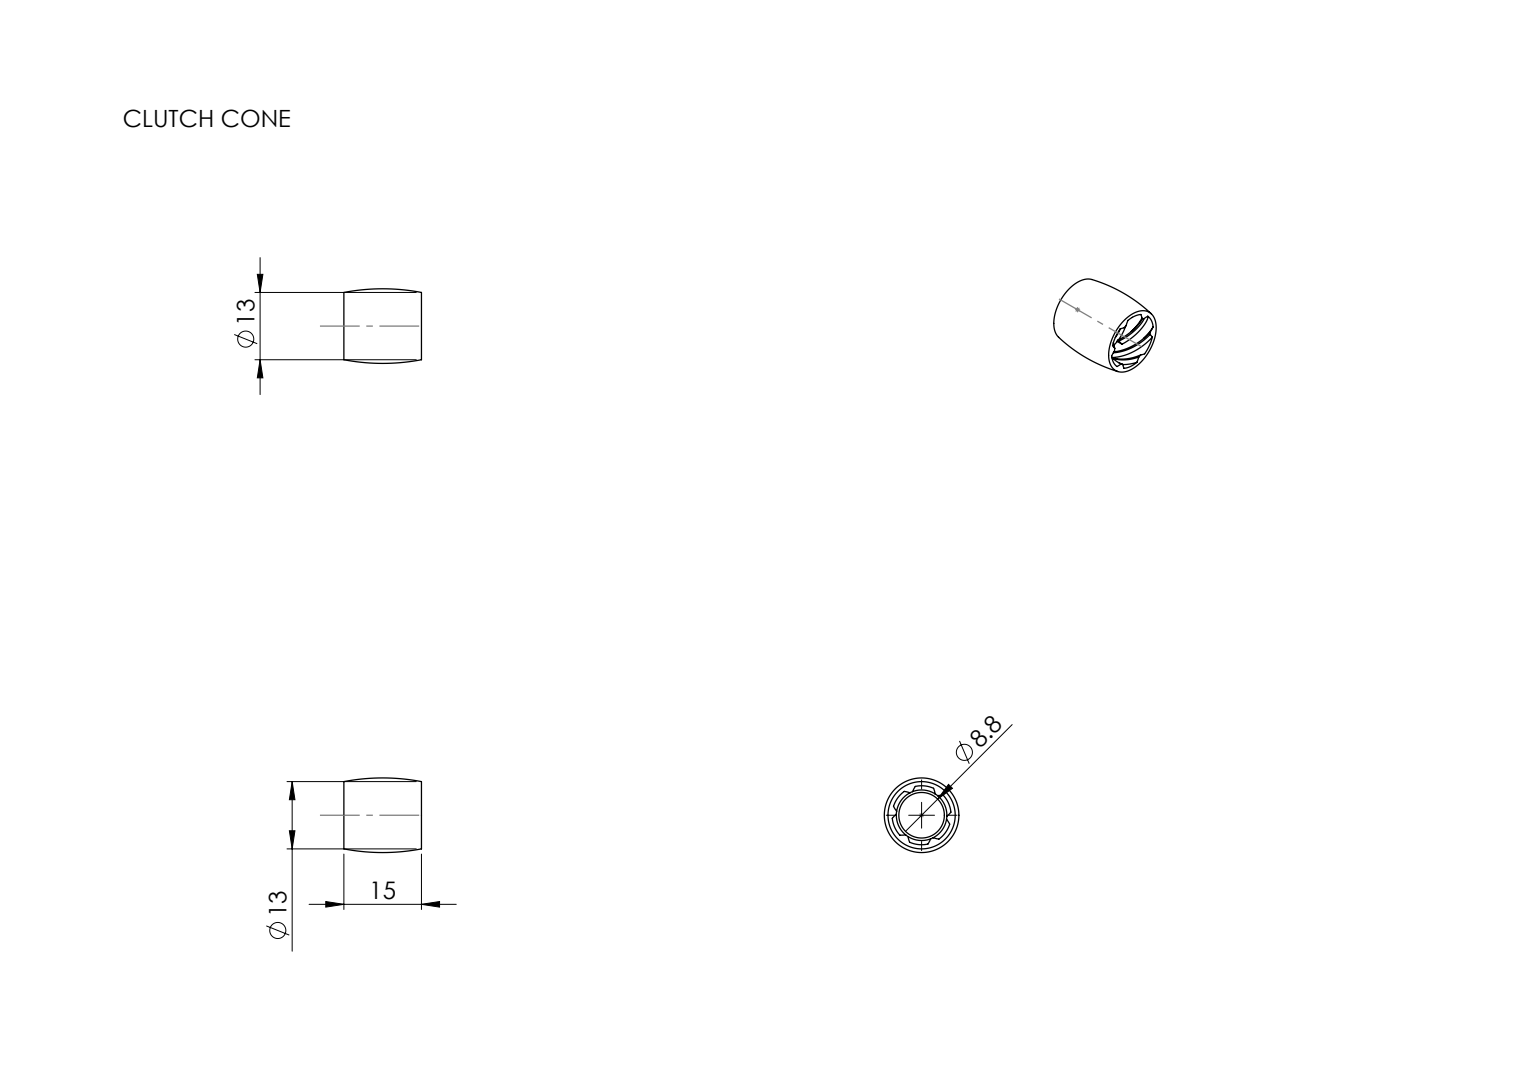
ISO-10303-21;
HEADER;
FILE_DESCRIPTION (('STEP AP214'),
    '1' );
FILE_NAME ('CLUTCH CONE.step',
    '2026-10-08T05:56:58',
    ( '' ),
    ( '' ),
    'SwSTEP 2.0',
    'SolidWorks 2026',
    '' );
FILE_SCHEMA (( 'AUTOMOTIVE_DESIGN' ));
ENDSEC;

DATA;
#4=FACE_OUTER_BOUND ( 'NONE', #5916, .T. ) ;
#7=CARTESIAN_POINT ( 'NONE',  ( 9.343749997951615427, -3.499494075959840966, 3.499494075959791672 ) ) ;
#8=EDGE_CURVE ( 'NONE', #13643, #9700, #6131, .T. ) ;
#15=VERTEX_POINT ( 'NONE', #17446 ) ;
#18=CARTESIAN_POINT ( 'NONE',  ( 12.84374999795161543, 1.016293382781411792, 4.781284448697195266 ) ) ;
#56=CARTESIAN_POINT ( 'NONE',  ( 12.34374999795161543, 4.888101187500000222, 0.7741991708318884946 ) ) ;
#57=ORIENTED_EDGE ( 'NONE', *, *, #11077, .F. ) ;
#63=CIRCLE ( 'NONE', #5149, 40.00000000000000711 ) ;
#70=ORIENTED_EDGE ( 'NONE', *, *, #8344, .T. ) ;
#73=DIRECTION ( 'NONE',  ( -1.000000000000000000, 0.000000000000000000, 0.000000000000000000 ) ) ;
#91=CARTESIAN_POINT ( 'NONE',  ( 13.34374999795161365, -0.2590123213420631454, -4.942249507334558700 ) ) ;
#94=CARTESIAN_POINT ( 'NONE',  ( 8.468749997951615427, -1.988169868018530462, -4.465502636338051445 ) ) ;
#100=AXIS2_PLACEMENT_3D ( 'NONE', #5188, #8093, #8295 ) ;
#103=CARTESIAN_POINT ( 'NONE',  ( -2.000000000000001776, 3.950217066951266176, 3.681818181818181213 ) ) ;
#104=CARTESIAN_POINT ( 'NONE',  ( 11.46874999795161543, -2.444050593750019651, 4.233219804643871598 ) ) ;
#105=CARTESIAN_POINT ( 'NONE',  ( 10.50000000000000711, 3.631840208645794821, 4.484949146646379781 ) ) ;
#106=FACE_OUTER_BOUND ( 'NONE', #19772, .T. ) ;
#139=AXIS2_PLACEMENT_3D ( 'NONE', #2060, #12472, #13976 ) ;
#145=ORIENTED_EDGE ( 'NONE', *, *, #8344, .F. ) ;
#146=CARTESIAN_POINT ( 'NONE',  ( 13.00000000000000533, 0.5958122406256767256, -5.668774803599153422 ) ) ;
#147=CARTESIAN_POINT ( 'NONE',  ( 10.34374999795161543, 0.2590123213421660631, -4.942249507334553371 ) ) ;
#148=ORIENTED_EDGE ( 'NONE', *, *, #16940, .F. ) ;
#156=( BOUNDED_SURFACE ( )  B_SPLINE_SURFACE ( 1, 2, ( 
 ( #19696, #12102, #10210, #2584, #16407, #18204, #1100, #2682, #8800, #7272, #189, #18685, #7680, #9499, #382, #3485, #10992 ),
 ( #15499, #9592, #10894, #9295, #13794, #4787, #17096, #10700, #6275, #4590, #15690, #10794, #17000, #15330, #18396, #284, #6461 ) ),
 .UNSPECIFIED., .F., .F., .F. ) 
 B_SPLINE_SURFACE_WITH_KNOTS ( ( 2, 2 ),
 ( 3, 2, 2, 2, 2, 2, 2, 2, 3 ),
 ( 0.000000000000000000, 1.000000000000000000 ),
 ( 0.000000000000000000, 0.05000000000000000278, 0.1000000000000000056, 0.1499999999999999944, 0.2000000000000000111, 0.2500000000000000000, 0.2999999999999999889, 0.3499999999999999778, 0.4000000000000000222 ),
 .UNSPECIFIED. ) 
 GEOMETRIC_REPRESENTATION_ITEM ( )  RATIONAL_B_SPLINE_SURFACE ( (
 ( 1.000000000000000000, 0.9876883405951377704, 1.000000000000000000, 0.9876883405951377704, 1.000000000000000000, 0.9876883405951377704, 1.000000000000000000, 0.9876883405951377704, 1.000000000000000000, 0.9876883405951377704, 1.000000000000000000, 0.9876883405951377704, 1.000000000000000000, 0.9876883405951377704, 1.000000000000000000, 0.9876883405951377704, 1.000000000000000000),
 ( 1.000000000000000000, 0.9876883405951377704, 1.000000000000000000, 0.9876883405951377704, 1.000000000000000000, 0.9876883405951377704, 1.000000000000000000, 0.9876883405951377704, 1.000000000000000000, 0.9876883405951377704, 1.000000000000000000, 0.9876883405951377704, 1.000000000000000000, 0.9876883405951377704, 1.000000000000000000, 0.9876883405951377704, 1.000000000000000000) ) ) 
 REPRESENTATION_ITEM ( '' )  SURFACE ( )  );
#174=EDGE_CURVE ( 'NONE', #16744, #5554, #14796, .T. ) ;
#175=CARTESIAN_POINT ( 'NONE',  ( 6.234374998975811266, 0.000000000000000000, -5.294050593750000644 ) ) ;
#186=CARTESIAN_POINT ( 'NONE',  ( 7.843749997951614539, -3.270778111535287191, -3.632567103900569361 ) ) ;
#189=CARTESIAN_POINT ( 'NONE',  ( 11.46874999795161543, 2.444050593750049405, -4.233219804643852946 ) ) ;
#193=AXIS2_PLACEMENT_3D ( 'NONE', #6002, #12326, #18419 ) ;
#203=CARTESIAN_POINT ( 'NONE',  ( 13.46874999795161543, -4.465502636338038123, 1.988169868018562880 ) ) ;
#210=CARTESIAN_POINT ( 'NONE',  ( -2.000000000000001776, 3.218695387886217674, 2.999999999999999556 ) ) ;
#211=AXIS2_PLACEMENT_3D ( 'NONE', #17804, #14615, #6883 ) ;
#213=CARTESIAN_POINT ( 'NONE',  ( 14.84374999795161543, -2.873153789725797935, -3.954556930911881096 ) ) ;
#243=CARTESIAN_POINT ( 'NONE',  ( 8.843749997951615427, -1.988169868018530462, -4.465502636338051445 ) ) ;
#252=CARTESIAN_POINT ( 'NONE',  ( 11.46874999795161543, 2.444050593749990785, 4.233219804643887585 ) ) ;
#284=CARTESIAN_POINT ( 'NONE',  ( 13.50000000000000533, 5.574407415329178939, -1.493657965219446382 ) ) ;
#289=CARTESIAN_POINT ( 'NONE',  ( 2.999999999999998224, -2.487173708821168283, 2.318181818181817455 ) ) ;
#299=CARTESIAN_POINT ( 'NONE',  ( 7.312499995903225525, 4.936344801571308061, -2.849999999999989431 ) ) ;
#308=CARTESIAN_POINT ( 'NONE',  ( 8.500000000000005329, -1.493657965219446160, -5.574407415329178939 ) ) ;
#320=ORIENTED_EDGE ( 'NONE', *, *, #14476, .T. ) ;
#343=CYLINDRICAL_SURFACE ( 'NONE', #4937, 5.400000000000000355 ) ;
#345=CARTESIAN_POINT ( 'NONE',  ( 6.843749997951615427, -3.413342815706642518E-14, 4.888101187500000222 ) ) ;
#346=CARTESIAN_POINT ( 'NONE',  ( 14.34374999795161365, -1.280903732194453859, 4.780397808154257078 ) ) ;
#379=CARTESIAN_POINT ( 'NONE',  ( 7.343749997951615427, -0.7741991708319229115, 4.888101187499994893 ) ) ;
#381=ORIENTED_EDGE ( 'NONE', *, *, #16041, .F. ) ;
#382=CARTESIAN_POINT ( 'NONE',  ( 13.46874999795161543, 4.465502636338051445, -1.988169868018530906 ) ) ;
#400=CARTESIAN_POINT ( 'NONE',  ( 6.468749997951615427, 4.233219804643887585, -2.444050593749990341 ) ) ;
#406=EDGE_LOOP ( 'NONE', ( #6297, #10419, #12416, #16842 ) ) ;
#407=CARTESIAN_POINT ( 'NONE',  ( 12.84374999795161543, -4.648860486681943627, -1.510506337161893642 ) ) ;
#416=CARTESIAN_POINT ( 'NONE',  ( 7.312499995903225525, 0.000000000000000000, -5.700000000000001066 ) ) ;
#418=PLANE ( 'NONE',  #2750 ) ;
#448=CARTESIAN_POINT ( 'NONE',  ( 10.31249999590322552, -0.5958122406255588199, -5.668774803599165857 ) ) ;
#463=CARTESIAN_POINT ( 'NONE',  ( 8.968749997951613651, 1.280903732194420996, 4.780397808154265960 ) ) ;
#485=CARTESIAN_POINT ( 'NONE',  ( 12.46874999795161543, 3.632567103900569361, -3.270778111535288080 ) ) ;
#494=DIRECTION ( 'NONE',  ( 0.000000000000000000, 0.7315216790650493905, -0.6818181818181815457 ) ) ;
#496=CARTESIAN_POINT ( 'NONE',  ( 6.843749997951615427, 4.233219804643887585, -2.444050593749990785 ) ) ;
#509=CARTESIAN_POINT ( 'NONE',  ( 14.46874999795161720, -1.988169868018592856, 4.465502636338025688 ) ) ;
#534=EDGE_LOOP ( 'NONE', ( #18812, #9374, #9796, #10381, #12618, #14253, #16988, #12583 ) ) ;
#545=VECTOR ( 'NONE', #19579, 1000.000000000000000 ) ;
#554=CARTESIAN_POINT ( 'NONE',  ( 11.84374999795161365, 2.444050593750049405, -4.233219804643852946 ) ) ;
#555=CARTESIAN_POINT ( 'NONE',  ( 9.343749997951615427, 1.280903732194420996, 4.780397808154265960 ) ) ;
#560=FACE_OUTER_BOUND ( 'NONE', #8813, .T. ) ;
#564=CARTESIAN_POINT ( 'NONE',  ( 9.165444847914525184, 0.2987243419133224775, 5.700000000000001954 ) ) ;
#566=CARTESIAN_POINT ( 'NONE',  ( 9.968749997951615427, -0.2590123213421313686, 4.942249507334556036 ) ) ;
#582=CARTESIAN_POINT ( 'NONE',  ( -2.000000000000001776, 3.950217066951266176, 3.681818181818181213 ) ) ;
#588=DIRECTION ( 'NONE',  ( -1.000000000000000000, -0.000000000000000000, -0.000000000000000000 ) ) ;
#593=CARTESIAN_POINT ( 'NONE',  ( 6.656249997951614539, 4.233219804643887585, -2.444050593749990341 ) ) ;
#603=UNCERTAINTY_MEASURE_WITH_UNIT (LENGTH_MEASURE( 1.000000000000000082E-05 ), #7664, 'distance_accuracy_value', 'NONE');
#606=CARTESIAN_POINT ( 'NONE',  ( 11.46874999795161543, -2.444050593749961031, -4.233219804643904460 ) ) ;
#611=CARTESIAN_POINT ( 'NONE',  ( 11.50000000000000355, 3.631840208645857437, -4.484949146646330931 ) ) ;
#618=CARTESIAN_POINT ( 'NONE',  ( 11.31249999590322375, 5.421022142882375938, -1.761396867937200739 ) ) ;
#624=CARTESIAN_POINT ( 'NONE',  ( 6.968749997951614539, -0.7741991708319229115, 4.888101187499994893 ) ) ;
#629=FACE_BOUND ( 'NONE', #5913, .T. ) ;
#653=CARTESIAN_POINT ( 'NONE',  ( 8.843749997951615427, 1.988169868018562436, 4.465502636338039011 ) ) ;
#654=CARTESIAN_POINT ( 'NONE',  ( 14.46874999795161720, -1.988169868018592856, 4.465502636338025688 ) ) ;
#659=CARTESIAN_POINT ( 'NONE',  ( 13.00000000000000000, -4.125339889944092953, 2.622041954598548941 ) ) ;
#660=EDGE_CURVE ( 'NONE', #13507, #7007, #3581, .T. ) ;
#664=CIRCLE ( 'NONE', #18238, 5.700000000000001954 ) ;
#668=CARTESIAN_POINT ( 'NONE',  ( 13.46874999795161543, 0.5109457054262118714, -4.861323657744403448 ) ) ;
#675=( LENGTH_UNIT ( ) NAMED_UNIT ( * ) SI_UNIT ( .MILLI., .METRE. ) );
#682=EDGE_LOOP ( 'NONE', ( #3661, #6850, #15777, #2392 ) ) ;
#685=CARTESIAN_POINT ( 'NONE',  ( 13.00000000000000178, -4.444590484536226960, -2.035510078342938733 ) ) ;
#703=EDGE_CURVE ( 'NONE', #2779, #5327, #19540, .T. ) ;
#704=FACE_OUTER_BOUND ( 'NONE', #6201, .T. ) ;
#710=PLANE ( 'NONE',  #13946 ) ;
#713=EDGE_CURVE ( 'NONE', #18575, #7007, #1785, .T. ) ;
#720=VERTEX_POINT ( 'NONE', #3211 ) ;
#752=ORIENTED_EDGE ( 'NONE', *, *, #660, .F. ) ;
#754=CARTESIAN_POINT ( 'NONE',  ( 13.00000000000000178, -4.920309236097862637, -1.604440756441545268 ) ) ;
#762=CARTESIAN_POINT ( 'NONE',  ( 12.65441706489329299, -5.699999999999998401, -0.6173595171471657483 ) ) ;
#781=CARTESIAN_POINT ( 'NONE',  ( 12.66727757604273386, -4.360680574150373717E-16, 5.700000000000001066 ) ) ;
#794=CARTESIAN_POINT ( 'NONE',  ( 10.34374999795161543, -4.150607464521772094, -2.695436003842760719 ) ) ;
#795=CARTESIAN_POINT ( 'NONE',  ( 9.312499995903225525, 2.318398865532038666, 5.207209108562838473 ) ) ;
#800=CIRCLE ( 'NONE', #3027, 6.500000000000002665 ) ;
#802=UNCERTAINTY_MEASURE_WITH_UNIT (LENGTH_MEASURE( 1.000000000000000082E-05 ), #13780, 'distance_accuracy_value', 'NONE');
#804=CARTESIAN_POINT ( 'NONE',  ( 13.84374999795161543, 0.5109457054262118714, -4.861323657744403448 ) ) ;
#808=LINE ( 'NONE', #16007, #5368 ) ;
#863=CARTESIAN_POINT ( 'NONE',  ( 7.000000000000005329, -1.761396867937238486, 5.421022142882364392 ) ) ;
#871=VERTEX_POINT ( 'NONE', #14621 ) ;
#878=CARTESIAN_POINT ( 'NONE',  ( 13.00000000000000178, -3.869963285057273605, 2.986818217332043446 ) ) ;
#887=CARTESIAN_POINT ( 'NONE',  ( 11.34374999795161543, 3.114526743279256049, 3.846120219227944670 ) ) ;
#897=AXIS2_PLACEMENT_3D ( 'NONE', #9316, #9724, #10914 ) ;
#902=CARTESIAN_POINT ( 'NONE',  ( 9.343749997951615427, -3.499494075959840966, 3.499494075959791672 ) ) ;
#914=EDGE_CURVE ( 'NONE', #11016, #5140, #8465, .T. ) ;
#917=( BOUNDED_CURVE ( )  B_SPLINE_CURVE ( 2, ( #9368, #13668, #1364, #16672, #9267, #19759, #1464, #6048, #12170, #18270, #4558, #56, #6149, #16875, #15372 ),
 .UNSPECIFIED., .F., .F. ) 
 B_SPLINE_CURVE_WITH_KNOTS ( ( 3, 2, 2, 2, 2, 2, 2, 3 ),
 ( 0.000000000000000000, 0.05000000000000000278, 0.1000000000000000056, 0.1499999999999999944, 0.2000000000000000111, 0.2500000000000000000, 0.2999999999999999889, 0.3078686208676164604 ),
 .UNSPECIFIED. ) 
 CURVE ( )  GEOMETRIC_REPRESENTATION_ITEM ( )  RATIONAL_B_SPLINE_CURVE ( ( 1.000000000000000000, 0.9876883405951377704, 1.000000000000000000, 0.9876883405951377704, 1.000000000000000000, 0.9876883405951377704, 1.000000000000000000, 0.9876883405951377704, 1.000000000000000000, 0.9876883405951377704, 1.000000000000000000, 0.9876883405951377704, 1.000000000000000000, 0.9980624843978382899, 0.9967347918236166837 ) ) 
 REPRESENTATION_ITEM ( '' )  );
#918=CARTESIAN_POINT ( 'NONE',  ( 9.312499995903225525, -5.668774803599153422, -0.5958122406256771697 ) ) ;
#939=ORIENTED_EDGE ( 'NONE', *, *, #8365, .F. ) ;
#964=CARTESIAN_POINT ( 'NONE',  ( 12.50000000000000533, -4.840010801796506890, 3.143139765844590983 ) ) ;
#976=CARTESIAN_POINT ( 'NONE',  ( 13.00000000000000178, 0.000000000000000000, 0.000000000000000000 ) ) ;
#979=EDGE_CURVE ( 'NONE', #11644, #4794, #11939, .T. ) ;
#1002=DIRECTION ( 'NONE',  ( 0.000000000000000000, 0.4999999999999920619, 0.8660254037844432595 ) ) ;
#1011=DIRECTION ( 'NONE',  ( -1.000000000000000000, 0.000000000000000000, 0.000000000000000000 ) ) ;
#1037=CARTESIAN_POINT ( 'NONE',  ( 11.96874999795161365, -3.114526743279282250, 3.846120219227923798 ) ) ;
#1067=CARTESIAN_POINT ( 'NONE',  ( 11.00000000000000711, -2.850000000000023626, 4.936344801571289409 ) ) ;
#1080=CARTESIAN_POINT ( 'NONE',  ( 12.84374999795161543, 4.648860486681953397, 1.510506337161861223 ) ) ;
#1081=CARTESIAN_POINT ( 'NONE',  ( 9.343749997951615427, 4.780397808154257078, 1.280903732194454081 ) ) ;
#1100=CARTESIAN_POINT ( 'NONE',  ( 9.468749997951615427, -0.5109457054261099529, -4.861323657744413218 ) ) ;
#1110=CARTESIAN_POINT ( 'NONE',  ( 10.00000000000000533, -5.421022142882388373, 1.761396867937162769 ) ) ;
#1114=CARTESIAN_POINT ( 'NONE',  ( 9.468749997951615427, -3.954556930911881985, 2.873153789725797491 ) ) ;
#1136=CARTESIAN_POINT ( 'NONE',  ( 13.00000000000000000, 1.727010089215937905, 5.432074755721460591 ) ) ;
#1139=CARTESIAN_POINT ( 'NONE',  ( 7.968749997951616315, 2.695436003842704764, 4.150607464521812062 ) ) ;
#1145=CARTESIAN_POINT ( 'NONE',  ( 8.500000000000007105, -5.574407415329147852, -1.493657965219562511 ) ) ;
#1148=EDGE_CURVE ( 'NONE', #5529, #11664, #6279, .T. ) ;
#1150=ADVANCED_FACE ( 'NONE', ( #6371 ), #5472, .F. ) ;
#1165=CARTESIAN_POINT ( 'NONE',  ( 11.50000000000000355, -3.631840208645826351, 4.484949146646356688 ) ) ;
#1166=CIRCLE ( 'NONE', #11076, 6.500000000000000000 ) ;
#1177=CARTESIAN_POINT ( 'NONE',  ( 11.31249999590322375, 5.421022142882375938, -1.761396867937200739 ) ) ;
#1184=DIRECTION ( 'NONE',  ( -1.000000000000000000, -0.000000000000000000, -0.000000000000000000 ) ) ;
#1190=CARTESIAN_POINT ( 'NONE',  ( 12.99999999999999467, 4.496324317583058949, 1.917446440021246756 ) ) ;
#1198=LINE ( 'NONE', #9203, #10258 ) ;
#1211=CARTESIAN_POINT ( 'NONE',  ( 12.84374999795161543, 4.648860486681953397, 1.510506337161861223 ) ) ;
#1217=CARTESIAN_POINT ( 'NONE',  ( 11.31249999590322375, -1.185096637661254171, 5.575441324182689229 ) ) ;
#1236=CARTESIAN_POINT ( 'NONE',  ( 11.46874999795161543, -2.444050593749961031, -4.233219804643904460 ) ) ;
#1247=EDGE_CURVE ( 'NONE', #19695, #4381, #18662, .T. ) ;
#1253=CARTESIAN_POINT ( 'NONE',  ( 12.73273607671833929, -0.6164700669140440459, -4.866269517993464078 ) ) ;
#1263=CARTESIAN_POINT ( 'NONE',  ( 9.000000000000005329, 0.5958122406255991210, 5.668774803599163192 ) ) ;
#1270=EDGE_LOOP ( 'NONE', ( #9959, #8302, #10280, #10813 ) ) ;
#1275=CARTESIAN_POINT ( 'NONE',  ( -2.000000000000001776, -3.950217066951263956, -3.681818181818183877 ) ) ;
#1293=CARTESIAN_POINT ( 'NONE',  ( 7.343749997951615427, 3.846120219227923798, 3.114526743279282694 ) ) ;
#1297=CARTESIAN_POINT ( 'NONE',  ( 13.00000000000000178, 0.000000000000000000, 0.000000000000000000 ) ) ;
#1298=CARTESIAN_POINT ( 'NONE',  ( 12.00000000000000533, 1.185096637661215757, 5.575441324182695446 ) ) ;
#1300=CARTESIAN_POINT ( 'NONE',  ( 11.46874999795161543, 4.888101187500000222, -2.993098736590125853E-16 ) ) ;
#1305=CARTESIAN_POINT ( 'NONE',  ( 13.00000000000000000, -1.727010089215899713, -5.432074755721473025 ) ) ;
#1306=EDGE_LOOP ( 'NONE', ( #18307, #12651, #14806, #1467 ) ) ;
#1309=CARTESIAN_POINT ( 'NONE',  ( 9.343749997951615427, 3.499494075959816541, -3.499494075959816541 ) ) ;
#1312=CARTESIAN_POINT ( 'NONE',  ( 6.234374998975811266, -3.696815770993907903E-14, 5.294050593750000644 ) ) ;
#1319=CARTESIAN_POINT ( 'NONE',  ( -2.000000000000001776, 0.000000000000000000, 0.000000000000000000 ) ) ;
#1323=DIRECTION ( 'NONE',  ( 0.000000000000000000, 0.000000000000000000, 1.000000000000000000 ) ) ;
#1324=CARTESIAN_POINT ( 'NONE',  ( 11.96874999795161365, 4.888101187500000222, 0.7741991708318884946 ) ) ;
#1333=CARTESIAN_POINT ( 'NONE',  ( 14.46874999795161720, 1.988169868018623720, -4.465502636338010589 ) ) ;
#1334=VECTOR ( 'NONE', #5423, 1000.000000000000000 ) ;
#1347=CIRCLE ( 'NONE', #4219, 5.400000000000000355 ) ;
#1351=ADVANCED_FACE ( 'NONE', ( #10582 ), #7915, .F. ) ;
#1359=DIRECTION ( 'NONE',  ( -1.000000000000000000, 0.000000000000000000, 0.000000000000000000 ) ) ;
#1364=CARTESIAN_POINT ( 'NONE',  ( 7.843749997951614539, 1.510506337161861445, -4.648860486681953397 ) ) ;
#1370=AXIS2_PLACEMENT_3D ( 'NONE', #6319, #18637, #4934 ) ;
#1375=COLOUR_RGB ( '', 0.31764706, 0.68627451, 0.89019608) ;
#1388=PRODUCT_DEFINITION_CONTEXT ( 'detailed design', #10473, 'design' ) ;
#1398=ORIENTED_EDGE ( 'NONE', *, *, #1665, .T. ) ;
#1399=CARTESIAN_POINT ( 'NONE',  ( 11.34374999795161543, -1.773574444220757274, 4.620319390059819398 ) ) ;
#1402=AXIS2_PLACEMENT_3D ( 'NONE', #15006, #10704, #16607 ) ;
#1404=CARTESIAN_POINT ( 'NONE',  ( 10.50000000000000533, 3.631840208645794821, 4.484949146646379781 ) ) ;
#1408=DIRECTION ( 'NONE',  ( 0.000000000000000000, 0.000000000000000000, 1.000000000000000000 ) ) ;
#1427=CARTESIAN_POINT ( 'NONE',  ( 8.812499995903225525, 5.763142191869157216, -0.3020334839682480288 ) ) ;
#1438=CARTESIAN_POINT ( 'NONE',  ( 8.000000000000005329, -5.668774803599153422, -0.5958122406256771697 ) ) ;
#1442=( BOUNDED_CURVE ( )  B_SPLINE_CURVE ( 2, ( #19181, #2085, #15798, #15900, #795, #5474, #11300, #3588, #8495 ),
 .UNSPECIFIED., .F., .F. ) 
 B_SPLINE_CURVE_WITH_KNOTS ( ( 3, 2, 2, 2, 3 ),
 ( 0.000000000000000000, 0.04999999999999999584, 0.09999999999999999167, 0.1499999999999999944, 0.1666819079834116757 ),
 .UNSPECIFIED. ) 
 CURVE ( )  GEOMETRIC_REPRESENTATION_ITEM ( )  RATIONAL_B_SPLINE_CURVE ( ( 1.000000000000000000, 0.9876883405951377704, 1.000000000000000000, 0.9876883405951377704, 1.000000000000000000, 0.9876883405951377704, 1.000000000000000000, 0.9958923606136996787, 0.9945256517182512468 ) ) 
 REPRESENTATION_ITEM ( '' )  );
#1443=EDGE_CURVE ( 'NONE', #3546, #9343, #18377, .T. ) ;
#1446=CARTESIAN_POINT ( 'NONE',  ( 13.00000000000000178, 3.849641071994447383, -3.458892414715164065 ) ) ;
#1464=CARTESIAN_POINT ( 'NONE',  ( 9.843749997951615427, 3.954556930911862000, -2.873153789725825469 ) ) ;
#1467=ORIENTED_EDGE ( 'NONE', *, *, #6341, .F. ) ;
#1468=EDGE_CURVE ( 'NONE', #11673, #18486, #18038, .T. ) ;
#1473=CARTESIAN_POINT ( 'NONE',  ( 9.812499995903223748, 4.080749450109650844, -4.080749450109650844 ) ) ;
#1494=CARTESIAN_POINT ( 'NONE',  ( 12.34374999795161543, -3.114526743279282250, 3.846120219227923798 ) ) ;
#1497=CARTESIAN_POINT ( 'NONE',  ( -2.000000000000001776, 0.000000000000000000, 0.000000000000000000 ) ) ;
#1498=CARTESIAN_POINT ( 'NONE',  ( 12.33180101230371584, 0.5990941410143489909, 5.700000000000001066 ) ) ;
#1499=EDGE_CURVE ( 'NONE', #871, #3717, #6504, .T. ) ;
#1501=ORIENTED_EDGE ( 'NONE', *, *, #11729, .T. ) ;
#1507=CARTESIAN_POINT ( 'NONE',  ( 12.65441706489329299, -2.315350974882445456, -5.245024560144885939 ) ) ;
#1513=CARTESIAN_POINT ( 'NONE',  ( 12.46874999795161543, 4.648860486681953397, 1.510506337161861223 ) ) ;
#1517=ORIENTED_EDGE ( 'NONE', *, *, #3744, .F. ) ;
#1527=CARTESIAN_POINT ( 'NONE',  ( 9.312499995903225525, 5.668774803599156975, 0.5958122406256377568 ) ) ;
#1528=CARTESIAN_POINT ( 'NONE',  ( 13.00000000000000000, 4.333424887443004359, 2.261628166637590365 ) ) ;
#1538=CARTESIAN_POINT ( 'NONE',  ( 9.968749997951615427, 4.150607464521791634, 2.695436003842732298 ) ) ;
#1549=DIRECTION ( 'NONE',  ( -1.000000000000000000, -0.000000000000000000, -0.000000000000000000 ) ) ;
#1555=EDGE_CURVE ( 'NONE', #5021, #2350, #12018, .T. ) ;
#1569=CARTESIAN_POINT ( 'NONE',  ( 7.843749997951614539, 3.270778111535313837, 3.632567103900546712 ) ) ;
#1593=CARTESIAN_POINT ( 'NONE',  ( 6.500000000000005329, 5.387740456496234565, -2.068159791354182708 ) ) ;
#1595=EDGE_LOOP ( 'NONE', ( #18905, #4122 ) ) ;
#1596=CARTESIAN_POINT ( 'NONE',  ( 8.500000000000007105, 4.080749450109650844, -4.080749450109650844 ) ) ;
#1611=CARTESIAN_POINT ( 'NONE',  ( 9.968749997951617203, -4.409619785863921670, 2.246813503491803310 ) ) ;
#1620=CARTESIAN_POINT ( 'NONE',  ( 10.96874999795161720, 4.888101187500000222, -0.7741991708318890497 ) ) ;
#1630=DIRECTION ( 'NONE',  ( -1.000000000000000000, 0.000000000000000000, 0.000000000000000000 ) ) ;
#1631=CARTESIAN_POINT ( 'NONE',  ( 11.96874999795161365, 1.773574444220725299, 4.620319390059829168 ) ) ;
#1638=APPLICATION_CONTEXT ( 'automotive_design' ) ;
#1645=CARTESIAN_POINT ( 'NONE',  ( 9.343749997951615427, -1.280903732194386579, -4.780397808154273953 ) ) ;
#1647=ORIENTED_EDGE ( 'NONE', *, *, #11077, .T. ) ;
#1665=EDGE_CURVE ( 'NONE', #18575, #9272, #2209, .T. ) ;
#1669=CARTESIAN_POINT ( 'NONE',  ( 13.00000000000000178, -0.7793280607714923036, -4.825575716215948496 ) ) ;
#1718=ORIENTED_EDGE ( 'NONE', *, *, #4065, .T. ) ;
#1722=CARTESIAN_POINT ( 'NONE',  ( 13.00000000000000000, 5.567819778318904511, 1.220402768007685657 ) ) ;
#1736=CARTESIAN_POINT ( 'NONE',  ( 13.00000000000000000, 0.2080849974989116558, 4.883670121236158401 ) ) ;
#1747=CARTESIAN_POINT ( 'NONE',  ( 11.81249999590322552, 2.068159791354259092, -5.387740456496206143 ) ) ;
#1755=CARTESIAN_POINT ( 'NONE',  ( 12.84374999795161543, 1.016293382781411792, 4.781284448697194378 ) ) ;
#1785=( BOUNDED_CURVE ( )  B_SPLINE_CURVE ( 2, ( #416, #3613, #6496, #12425, #15721, #12625, #17320, #14321, #618, #6694, #3511, #17222, #11325 ),
 .UNSPECIFIED., .F., .F. ) 
 B_SPLINE_CURVE_WITH_KNOTS ( ( 3, 2, 2, 2, 2, 2, 3 ),
 ( 0.000000000000000000, 0.05000000000000000278, 0.1000000000000000056, 0.1499999999999999944, 0.2000000000000000111, 0.2500000000000000000, 0.2843253191101273170 ),
 .UNSPECIFIED. ) 
 CURVE ( )  GEOMETRIC_REPRESENTATION_ITEM ( )  RATIONAL_B_SPLINE_CURVE ( ( 1.000000000000000000, 0.9876883405951377704, 1.000000000000000000, 0.9876883405951377704, 1.000000000000000000, 0.9876883405951377704, 1.000000000000000000, 0.9876883405951377704, 1.000000000000000000, 0.9876883405951377704, 1.000000000000000000, 0.9915479672430580482, 0.9947006833465674713 ) ) 
 REPRESENTATION_ITEM ( '' )  );
#1786=CARTESIAN_POINT ( 'NONE',  ( 9.843749997951615427, -4.465502636338009701, -1.988169868018624609 ) ) ;
#1800=CARTESIAN_POINT ( 'NONE',  ( 9.000000000000005329, 5.207209108562820710, 2.318398865532074193 ) ) ;
#1809=CARTESIAN_POINT ( 'NONE',  ( 11.46874999795161543, -4.888101187500000222, -3.383411828340740850E-14 ) ) ;
#1815=EDGE_LOOP ( 'NONE', ( #19167, #8420, #70, #12884 ) ) ;
#1852=CARTESIAN_POINT ( 'NONE',  ( 8.843749997951615427, 4.861323657744407001, 0.5109457054261784537 ) ) ;
#1853=VERTEX_POINT ( 'NONE', #14815 ) ;
#1876=CARTESIAN_POINT ( 'NONE',  ( 12.99999999999999467, 4.057257337410506537, -2.726922038711639740 ) ) ;
#1878=EDGE_LOOP ( 'NONE', ( #6627, #4972, #13147, #5239, #9251 ) ) ;
#1884=CARTESIAN_POINT ( 'NONE',  ( 11.34374999795161543, -3.114526743279228072, -3.846120219227966430 ) ) ;
#1903=DIRECTION ( 'NONE',  ( 0.000000000000000000, 0.000000000000000000, -1.000000000000000000 ) ) ;
#1937=CARTESIAN_POINT ( 'NONE',  ( 14.31249999590322552, 5.207209108562852684, -2.318398865532001363 ) ) ;
#1943=CARTESIAN_POINT ( 'NONE',  ( 12.96874999795161543, 0.2590123213420971182, 4.942249507334556924 ) ) ;
#1973=ORIENTED_EDGE ( 'NONE', *, *, #10065, .T. ) ;
#1974=CARTESIAN_POINT ( 'NONE',  ( 13.34374999795161365, 4.150607464521828938, -2.695436003842674566 ) ) ;
#2000=ORIENTED_EDGE ( 'NONE', *, *, #14470, .F. ) ;
#2006=CARTESIAN_POINT ( 'NONE',  ( 11.00000000000000711, 2.850000000000057820, -4.936344801571268093 ) ) ;
#2028=VERTEX_POINT ( 'NONE', #13504 ) ;
#2038=CARTESIAN_POINT ( 'NONE',  ( 10.81249999590322375, 0.3020334839683282979, -5.763142191869152775 ) ) ;
#2039=CARTESIAN_POINT ( 'NONE',  ( 13.00000000000000178, -0.7156116249825553721, -4.835865888676779356 ) ) ;
#2046=CARTESIAN_POINT ( 'NONE',  ( 6.000000000000005329, 0.000000000000000000, 0.000000000000000000 ) ) ;
#2060=CARTESIAN_POINT ( 'NONE',  ( 13.00000000000000178, 4.400000000000000355, 0.000000000000000000 ) ) ;
#2075=( BOUNDED_CURVE ( )  B_SPLINE_CURVE ( 2, ( #3081, #19596, #10698 ),
 .UNSPECIFIED., .F., .F. ) 
 B_SPLINE_CURVE_WITH_KNOTS ( ( 3, 3 ),
 ( 0.3333180920165871863, 0.3500000000000000333 ),
 .UNSPECIFIED. ) 
 CURVE ( )  GEOMETRIC_REPRESENTATION_ITEM ( )  RATIONAL_B_SPLINE_CURVE ( ( 0.9945256517182510247, 0.9958923606136993456, 1.000000000000000000 ) ) 
 REPRESENTATION_ITEM ( '' )  );
#2079=CARTESIAN_POINT ( 'NONE',  ( 9.000000000000005329, 4.611396867937201272, -3.350375938067097437 ) ) ;
#2085=CARTESIAN_POINT ( 'NONE',  ( 7.812499995903224637, 4.484949146646356688, 3.631840208645826795 ) ) ;
#2094=CARTESIAN_POINT ( 'NONE',  ( 10.96874999795161720, -1.773574444220757274, 4.620319390059819398 ) ) ;
#2101=CARTESIAN_POINT ( 'NONE',  ( 9.843749997951615427, -3.954556930911881985, 2.873153789725797491 ) ) ;
#2143=ORIENTED_EDGE ( 'NONE', *, *, #2952, .T. ) ;
#2144=CARTESIAN_POINT ( 'NONE',  ( 6.468749997951615427, 4.233219804643887585, -2.444050593749990341 ) ) ;
#2159=VECTOR ( 'NONE', #8743, 1000.000000000000000 ) ;
#2164=DIRECTION ( 'NONE',  ( -1.000000000000000000, -0.000000000000000000, -0.000000000000000000 ) ) ;
#2169=CARTESIAN_POINT ( 'NONE',  ( 12.99999999999999467, 3.985098679772364427, -2.831373229855470797 ) ) ;
#2174=CARTESIAN_POINT ( 'NONE',  ( 8.468749997951615427, -1.988169868018530462, -4.465502636338051445 ) ) ;
#2175=CARTESIAN_POINT ( 'NONE',  ( 12.31249999590322552, 2.850000000000057820, -4.936344801571268093 ) ) ;
#2184=CARTESIAN_POINT ( 'NONE',  ( -2.000000000000001776, 0.000000000000000000, 0.000000000000000000 ) ) ;
#2195=CARTESIAN_POINT ( 'NONE',  ( 13.84374999795161543, -3.954556930911842016, -2.873153789725852558 ) ) ;
#2209=LINE ( 'NONE', #18820, #15168 ) ;
#2211=CARTESIAN_POINT ( 'NONE',  ( 6.468749997951615427, -3.413342815706642518E-14, 4.888101187500000222 ) ) ;
#2243=CARTESIAN_POINT ( 'NONE',  ( 13.34374999795161365, -4.150607464521812062, 2.695436003842704764 ) ) ;
#2264=VECTOR ( 'NONE', #14846, 1000.000000000000114 ) ;
#2265=FILL_AREA_STYLE_COLOUR ( '', #1375 ) ;
#2274=CARTESIAN_POINT ( 'NONE',  ( 7.968749997951616315, -2.695436003842674566, -4.150607464521828938 ) ) ;
#2275=CARTESIAN_POINT ( 'NONE',  ( 9.843749997951615427, -0.5109457054261099529, -4.861323657744413218 ) ) ;
#2279=CARTESIAN_POINT ( 'NONE',  ( 10.50000000000000533, 5.700000000000000178, -0.9027913098498572264 ) ) ;
#2292=CARTESIAN_POINT ( 'NONE',  ( 8.843749997951615427, -4.861323657744403448, -0.5109457054262123155 ) ) ;
#2297=CARTESIAN_POINT ( 'NONE',  ( 12.00000000000000533, 4.235925505221192822, -3.814044456245444081 ) ) ;
#2306=ORIENTED_EDGE ( 'NONE', *, *, #1555, .T. ) ;
#2314=DIRECTION ( 'NONE',  ( 1.000000000000000000, 0.000000000000000000, 0.000000000000000000 ) ) ;
#2350=VERTEX_POINT ( 'NONE', #19088 ) ;
#2357=PLANE ( 'NONE',  #12766 ) ;
#2363=SURFACE_STYLE_USAGE ( .BOTH. , #12875 ) ;
#2371=CARTESIAN_POINT ( 'NONE',  ( 12.34374999795161543, 3.114526743279308896, -3.846120219227901593 ) ) ;
#2372=CARTESIAN_POINT ( 'NONE',  ( 11.31249999590322375, 1.185096637661293251, -5.575441324182679459 ) ) ;
#2384=CARTESIAN_POINT ( 'NONE',  ( 10.81249999590322375, 4.840010801796482909, 3.143139765844622957 ) ) ;
#2385=CIRCLE ( 'NONE', #18054, 5.400000000000000355 ) ;
#2389=CARTESIAN_POINT ( 'NONE',  ( 10.34374999795161543, -4.150607464521772094, -2.695436003842760275 ) ) ;
#2392=ORIENTED_EDGE ( 'NONE', *, *, #6340, .F. ) ;
#2393=CARTESIAN_POINT ( 'NONE',  ( 15.31249999590322552, -3.350375938067065906, -4.611396867937224364 ) ) ;
#2417=DIRECTION ( 'NONE',  ( 0.000000000000000000, 0.000000000000000000, 1.000000000000000000 ) ) ;
#2422=AXIS2_PLACEMENT_3D ( 'NONE', #19522, #10438, #1323 ) ;
#2442=ORIENTED_EDGE ( 'NONE', *, *, #14853, .T. ) ;
#2445=CARTESIAN_POINT ( 'NONE',  ( 13.00000000000000533, -4.611396867937178179, -3.350375938067128967 ) ) ;
#2451=FILL_AREA_STYLE ('',( #2265 ) ) ;
#2456=CARTESIAN_POINT ( 'NONE',  ( 9.968749997951617203, -0.2590123213421313686, 4.942249507334556036 ) ) ;
#2461=CARTESIAN_POINT ( 'NONE',  ( 6.843749997951615427, -4.233219804643852946, -2.444050593750049849 ) ) ;
#2476=CARTESIAN_POINT ( 'NONE',  ( 11.31249999590322375, 4.235925505221138643, 3.814044456245502701 ) ) ;
#2480=EDGE_CURVE ( 'NONE', #18417, #2569, #18920, .T. ) ;
#2485=DIRECTION ( 'NONE',  ( 1.000000000000000000, 0.000000000000000000, 0.000000000000000000 ) ) ;
#2490=CARTESIAN_POINT ( 'NONE',  ( -2.000000000000001776, 5.388445916248354013E-16, -4.400000000000000355 ) ) ;
#2530=CARTESIAN_POINT ( 'NONE',  ( -2.000000000000001776, 0.000000000000000000, 0.000000000000000000 ) ) ;
#2533=CARTESIAN_POINT ( 'NONE',  ( 9.000000000000005329, 0.5958122406255991210, 5.668774803599163192 ) ) ;
#2536=EDGE_CURVE ( 'NONE', #5021, #18417, #18673, .T. ) ;
#2541=DIRECTION ( 'NONE',  ( -1.000000000000000000, -0.000000000000000000, -0.000000000000000000 ) ) ;
#2554=FACE_OUTER_BOUND ( 'NONE', #14176, .T. ) ;
#2555=ORIENTED_EDGE ( 'NONE', *, *, #18715, .T. ) ;
#2559=CARTESIAN_POINT ( 'NONE',  ( 7.312499995903225525, -4.936344801571268093, -2.850000000000058265 ) ) ;
#2569=VERTEX_POINT ( 'NONE', #11075 ) ;
#2584=CARTESIAN_POINT ( 'NONE',  ( 7.968749997951616315, -2.695436003842674566, -4.150607464521828938 ) ) ;
#2607=CARTESIAN_POINT ( 'NONE',  ( 2.999999999999998224, 0.000000000000000000, 0.000000000000000000 ) ) ;
#2627=CARTESIAN_POINT ( 'NONE',  ( 2.999999999999998224, 3.950217066951266176, 3.681818181818181213 ) ) ;
#2631=CARTESIAN_POINT ( 'NONE',  ( 2.999999999999998224, -3.950217066951263956, -3.681818181818183877 ) ) ;
#2632=ORIENTED_EDGE ( 'NONE', *, *, #10042, .T. ) ;
#2634=MANIFOLD_SOLID_BREP ( 'Cut-Extrude-Thin1', #18032 ) ;
#2650=ORIENTED_EDGE ( 'NONE', *, *, #14058, .F. ) ;
#2660=VERTEX_POINT ( 'NONE', #18973 ) ;
#2681=EDGE_LOOP ( 'NONE', ( #14546, #4895, #5342, #15515 ) ) ;
#2682=CARTESIAN_POINT ( 'NONE',  ( 9.968749997951617203, 0.2590123213421660631, -4.942249507334553371 ) ) ;
#2685=CARTESIAN_POINT ( 'NONE',  ( 8.312499995903225525, -5.575441324182703440, 1.185096637661176677 ) ) ;
#2686=CARTESIAN_POINT ( 'NONE',  ( 13.00000000000000178, 0.000000000000000000, 6.500000000000002665 ) ) ;
#2688=EDGE_CURVE ( 'NONE', #16413, #17466, #13505, .T. ) ;
#2700=CARTESIAN_POINT ( 'NONE',  ( 9.968749997951617203, 4.409619785863906571, -2.246813503491833508 ) ) ;
#2703=ORIENTED_EDGE ( 'NONE', *, *, #713, .T. ) ;
#2706=DIRECTION ( 'NONE',  ( -1.000000000000000000, 0.000000000000000000, 0.000000000000000000 ) ) ;
#2709=( BOUNDED_CURVE ( )  B_SPLINE_CURVE ( 2, ( #9967, #15865, #18957, #11646, #16253, #19245, #8551, #6837, #14465, #17561, #11365, #762, #14660 ),
 .UNSPECIFIED., .F., .F. ) 
 B_SPLINE_CURVE_WITH_KNOTS ( ( 3, 2, 2, 2, 2, 2, 3 ),
 ( 0.000000000000000000, 0.05000000000000000278, 0.1000000000000000056, 0.1499999999999999944, 0.2000000000000000111, 0.2500000000000000000, 0.2843253191101272614 ),
 .UNSPECIFIED. ) 
 CURVE ( )  GEOMETRIC_REPRESENTATION_ITEM ( )  RATIONAL_B_SPLINE_CURVE ( ( 1.000000000000000000, 0.9876883405951377704, 1.000000000000000000, 0.9876883405951377704, 1.000000000000000000, 0.9876883405951377704, 1.000000000000000000, 0.9876883405951377704, 1.000000000000000000, 0.9876883405951377704, 1.000000000000000000, 0.9915479672430580482, 0.9947006833465674713 ) ) 
 REPRESENTATION_ITEM ( '' )  );
#2716=FACE_OUTER_BOUND ( 'NONE', #11184, .T. ) ;
#2717=CARTESIAN_POINT ( 'NONE',  ( 11.84374999795161365, -2.444050593750019651, 4.233219804643871598 ) ) ;
#2728=CARTESIAN_POINT ( 'NONE',  ( 7.500000000000005329, -5.763142191869158992, 0.3020334839682081163 ) ) ;
#2729=DIRECTION ( 'NONE',  ( 0.000000000000000000, 0.7315216790650492795, 0.6818181818181815457 ) ) ;
#2730=VERTEX_POINT ( 'NONE', #8864 ) ;
#2750=AXIS2_PLACEMENT_3D ( 'NONE', #17427, #1002, #14528 ) ;
#2751=CARTESIAN_POINT ( 'NONE',  ( 7.968749997951616315, 2.695436003842704764, 4.150607464521812062 ) ) ;
#2756=ORIENTED_EDGE ( 'NONE', *, *, #12082, .T. ) ;
#2759=EDGE_LOOP ( 'NONE', ( #5210, #19294, #7443, #4978 ) ) ;
#2764=CARTESIAN_POINT ( 'NONE',  ( 13.84374999795161543, 3.954556930911862000, 2.873153789725825025 ) ) ;
#2778=AXIS2_PLACEMENT_3D ( 'NONE', #14754, #13058, #2729 ) ;
#2779=VERTEX_POINT ( 'NONE', #4953 ) ;
#2784=CARTESIAN_POINT ( 'NONE',  ( 8.843749997951615427, 1.988169868018562436, 4.465502636338039011 ) ) ;
#2786=CARTESIAN_POINT ( 'NONE',  ( 6.656249997951614539, 4.936344801571289409, 2.850000000000024070 ) ) ;
#2787=CARTESIAN_POINT ( 'NONE',  ( 13.00000000000000000, 4.125339889944109828, -2.622041954598519187 ) ) ;
#2794=CARTESIAN_POINT ( 'NONE',  ( 14.46874999795161720, -2.873153789725797935, -3.954556930911881096 ) ) ;
#2797=ORIENTED_EDGE ( 'NONE', *, *, #12498, .T. ) ;
#2799=DIRECTION ( 'NONE',  ( 0.000000000000000000, 5.329070518200751394E-15, 1.000000000000000000 ) ) ;
#2801=ADVANCED_FACE ( 'NONE', ( #18363 ), #16964, .F. ) ;
#2803=CARTESIAN_POINT ( 'NONE',  ( 12.99999999999998046, -4.467995623377355230, -2.612285395956023493 ) ) ;
#2817=EDGE_LOOP ( 'NONE', ( #12909, #6116, #11935, #9643 ) ) ;
#2820=AXIS2_PLACEMENT_3D ( 'NONE', #5950, #18174, #8662 ) ;
#2821=CARTESIAN_POINT ( 'NONE',  ( 6.468749997951615427, 4.233219804643871598, 2.444050593750020095 ) ) ;
#2823=CARTESIAN_POINT ( 'NONE',  ( 6.656249997951614539, -3.980288726281172656E-14, 5.700000000000001066 ) ) ;
#2827=CARTESIAN_POINT ( 'NONE',  ( 12.99999999999999112, 4.467995623377368553, 2.612285395955995515 ) ) ;
#2857=CARTESIAN_POINT ( 'NONE',  ( 13.00000000000000533, -5.207209108562836697, 2.318398865532038666 ) ) ;
#2859=VERTEX_POINT ( 'NONE', #345 ) ;
#2863=DIRECTION ( 'NONE',  ( -0.000000000000000000, 0.8660254037844329345, 0.5000000000000097700 ) ) ;
#2865=CARTESIAN_POINT ( 'NONE',  ( 9.343749997951615427, 3.499494075959816541, -3.499494075959816541 ) ) ;
#2884=CARTESIAN_POINT ( 'NONE',  ( 12.84374999795161543, -3.632567103900546712, 3.270778111535314281 ) ) ;
#2887=CARTESIAN_POINT ( 'NONE',  ( 11.46874999795161543, 2.444050593750049405, -4.233219804643852946 ) ) ;
#2896=DIRECTION ( 'NONE',  ( 0.000000000000000000, 0.000000000000000000, 1.000000000000000000 ) ) ;
#2911=CARTESIAN_POINT ( 'NONE',  ( 15.31249999590322552, -2.318398865532073305, 5.207209108562820710 ) ) ;
#2923=CARTESIAN_POINT ( 'NONE',  ( 10.96874999795161720, -3.114526743279228072, -3.846120219227966430 ) ) ;
#2924=VECTOR ( 'NONE', #15921, 1000.000000000000227 ) ;
#2926=CARTESIAN_POINT ( 'NONE',  ( 12.73273607671833929, 0.6164700669140775746, 4.866269517993460525 ) ) ;
#2929=FACE_OUTER_BOUND ( 'NONE', #10183, .T. ) ;
#2952=EDGE_CURVE ( 'NONE', #5462, #12828, #11482, .T. ) ;
#2971=ORIENTED_EDGE ( 'NONE', *, *, #9449, .T. ) ;
#2974=ORIENTED_EDGE ( 'NONE', *, *, #12220, .F. ) ;
#2984=ADVANCED_FACE ( 'NONE', ( #4041 ), #18155, .F. ) ;
#2988=CARTESIAN_POINT ( 'NONE',  ( 8.343749997951611874, 2.695436003842704764, 4.150607464521812062 ) ) ;
#2991=DIRECTION ( 'NONE',  ( 0.000000000000000000, 0.000000000000000000, 1.000000000000000000 ) ) ;
#3001=CARTESIAN_POINT ( 'NONE',  ( 11.96874999795161365, -4.888101187499994893, -0.7741991708319226895 ) ) ;
#3002=CARTESIAN_POINT ( 'NONE',  ( 14.34374999795161365, 3.499494075959816541, 3.499494075959815653 ) ) ;
#3016=CARTESIAN_POINT ( 'NONE',  ( 9.343749997951615427, 4.780397808154257078, 1.280903732194454081 ) ) ;
#3026=CARTESIAN_POINT ( 'NONE',  ( 9.968749997951617203, -4.150607464521772094, -2.695436003842760275 ) ) ;
#3027=AXIS2_PLACEMENT_3D ( 'NONE', #12052, #18154, #6128 ) ;
#3028=CARTESIAN_POINT ( 'NONE',  ( 12.46874999795161543, 1.016293382781411792, 4.781284448697194378 ) ) ;
#3031=CARTESIAN_POINT ( 'NONE',  ( 2.999999999999998224, 0.000000000000000000, 0.000000000000000000 ) ) ;
#3045=CARTESIAN_POINT ( 'NONE',  ( 9.968749997951615427, -4.150607464521772094, -2.695436003842760719 ) ) ;
#3054=ORIENTED_EDGE ( 'NONE', *, *, #14618, .T. ) ;
#3060=ADVANCED_FACE ( 'NONE', ( #6286 ), #12413, .T. ) ;
#3065=( BOUNDED_CURVE ( )  B_SPLINE_CURVE ( 2, ( #7755, #14363, #12763, #6838, #8155, #463, #14056, #566, #14262, #12861, #6536, #11366, #6635, #14466, #659 ),
 .UNSPECIFIED., .F., .F. ) 
 B_SPLINE_CURVE_WITH_KNOTS ( ( 3, 2, 2, 2, 2, 2, 2, 3 ),
 ( 0.000000000000000000, 0.05000000000000000278, 0.1000000000000000056, 0.1499999999999999944, 0.2000000000000000111, 0.2500000000000000000, 0.2999999999999999889, 0.3265529187307101844 ),
 .UNSPECIFIED. ) 
 CURVE ( )  GEOMETRIC_REPRESENTATION_ITEM ( )  RATIONAL_B_SPLINE_CURVE ( ( 1.000000000000000000, 0.9876883405951377704, 1.000000000000000000, 0.9876883405951377704, 1.000000000000000000, 0.9876883405951377704, 1.000000000000000000, 0.9876883405951377704, 1.000000000000000000, 0.9876883405951377704, 1.000000000000000000, 0.9876883405951377704, 1.000000000000000000, 0.9934617901676502383, 0.9938679225082089896 ) ) 
 REPRESENTATION_ITEM ( '' )  );
#3069=VERTEX_POINT ( 'NONE', #8739 ) ;
#3081=CARTESIAN_POINT ( 'NONE',  ( 12.66727757604273386, -4.360680574150373717E-16, 5.700000000000001066 ) ) ;
#3089=CARTESIAN_POINT ( 'NONE',  ( 7.968749997951616315, -2.695436003842674122, -4.150607464521828938 ) ) ;
#3092=CARTESIAN_POINT ( 'NONE',  ( 12.00000000000000533, 5.421022142882376826, 1.761396867937200073 ) ) ;
#3101=CARTESIAN_POINT ( 'NONE',  ( 9.500000000000003553, 4.840010801796480244, 3.143139765844623401 ) ) ;
#3103=CARTESIAN_POINT ( 'NONE',  ( 12.34374999795161543, 4.888101187500000222, 0.7741991708318884946 ) ) ;
#3110=CARTESIAN_POINT ( 'NONE',  ( 7.468749997951615427, -1.510506337161893864, 4.648860486681943627 ) ) ;
#3113=VECTOR ( 'NONE', #17109, 1000.000000000000114 ) ;
#3130=ADVANCED_FACE ( 'NONE', ( #7892 ), #14100, .F. ) ;
#3133=VECTOR ( 'NONE', #19416, 1000.000000000000000 ) ;
#3188=FACE_OUTER_BOUND ( 'NONE', #2681, .T. ) ;
#3191=CARTESIAN_POINT ( 'NONE',  ( 10.50000000000000711, 5.699999999999999289, -0.9027913098498572264 ) ) ;
#3206=CARTESIAN_POINT ( 'NONE',  ( 13.96874999795161365, -3.499494075959791672, -3.499494075959840078 ) ) ;
#3211=CARTESIAN_POINT ( 'NONE',  ( 2.999999999999998224, 3.950217066951266176, -3.681818181818181213 ) ) ;
#3213=ORIENTED_EDGE ( 'NONE', *, *, #9370, .T. ) ;
#3228=CARTESIAN_POINT ( 'NONE',  ( 12.99999999999999467, 0.3952618871915727916, 4.872094134945738730 ) ) ;
#3247=CARTESIAN_POINT ( 'NONE',  ( 6.843749997951615427, 4.233219804643887585, -2.444050593749990341 ) ) ;
#3256=VECTOR ( 'NONE', #6278, 1000.000000000000000 ) ;
#3265=ORIENTED_EDGE ( 'NONE', *, *, #4373, .F. ) ;
#3283=CARTESIAN_POINT ( 'NONE',  ( 8.343749997951613651, -2.246813503491864150, 4.409619785863891472 ) ) ;
#3284=ORIENTED_EDGE ( 'NONE', *, *, #9449, .F. ) ;
#3302=CARTESIAN_POINT ( 'NONE',  ( 8.968749997951611874, 4.780397808154257078, 1.280903732194454303 ) ) ;
#3309=CARTESIAN_POINT ( 'NONE',  ( 7.000000000000005329, -3.814044456245443193, -4.235925505221191933 ) ) ;
#3318=ADVANCED_FACE ( 'NONE', ( #17696 ), #3991, .F. ) ;
#3345=CARTESIAN_POINT ( 'NONE',  ( 7.500000000000005329, -5.763142191869158992, 0.3020334839682081163 ) ) ;
#3385=CARTESIAN_POINT ( 'NONE',  ( 11.34374999795161543, -4.888101187500005551, 0.7741991708318548548 ) ) ;
#3386=EDGE_LOOP ( 'NONE', ( #12658, #18758, #13143, #5921, #14658 ) ) ;
#3414=ORIENTED_EDGE ( 'NONE', *, *, #19473, .F. ) ;
#3415=LINE ( 'NONE', #8210, #2924 ) ;
#3444=CARTESIAN_POINT ( 'NONE',  ( 8.343749997951611874, -2.695436003842674566, -4.150607464521828938 ) ) ;
#3449=SHAPE_DEFINITION_REPRESENTATION ( #13226, #14878 ) ;
#3452=CARTESIAN_POINT ( 'NONE',  ( 10.96874999795161720, 3.114526743279255161, 3.846120219227944670 ) ) ;
#3481=( BOUNDED_CURVE ( )  B_SPLINE_CURVE ( 2, ( #10155, #8255, #18857, #16062, #5442, #4048, #2533, #564, #5248 ),
 .UNSPECIFIED., .F., .F. ) 
 B_SPLINE_CURVE_WITH_KNOTS ( ( 3, 2, 2, 2, 3 ),
 ( 0.000000000000000000, 0.04999999999999999584, 0.09999999999999999167, 0.1499999999999999944, 0.1666819079834116757 ),
 .UNSPECIFIED. ) 
 CURVE ( )  GEOMETRIC_REPRESENTATION_ITEM ( )  RATIONAL_B_SPLINE_CURVE ( ( 1.000000000000000000, 0.9876883405951377704, 1.000000000000000000, 0.9876883405951377704, 1.000000000000000000, 0.9876883405951377704, 1.000000000000000000, 0.9958923606136996787, 0.9945256517182512468 ) ) 
 REPRESENTATION_ITEM ( '' )  );
#3485=CARTESIAN_POINT ( 'NONE',  ( 13.96874999795161365, 4.780397808154273065, -1.280903732194386802 ) ) ;
#3499=CARTESIAN_POINT ( 'NONE',  ( 10.96874999795161720, 3.114526743279255161, 3.846120219227944670 ) ) ;
#3506=CARTESIAN_POINT ( 'NONE',  ( 12.96874999795161543, -4.409619785863891472, -2.246813503491864150 ) ) ;
#3511=CARTESIAN_POINT ( 'NONE',  ( 12.31249999590322552, 5.700000000000001066, -3.490243377569957047E-16 ) ) ;
#3525=DIRECTION ( 'NONE',  ( -0.000000000000000000, 0.6818181818181816567, 0.7315216790650493905 ) ) ;
#3537=DIRECTION ( 'NONE',  ( -1.000000000000000000, -0.000000000000000000, -0.000000000000000000 ) ) ;
#3538=CARTESIAN_POINT ( 'NONE',  ( 7.843749997951614539, -3.270778111535287191, -3.632567103900569361 ) ) ;
#3546=VERTEX_POINT ( 'NONE', #17235 ) ;
#3573=CARTESIAN_POINT ( 'NONE',  ( 12.96874999795161543, 4.150607464521828938, -2.695436003842674566 ) ) ;
#3575=CARTESIAN_POINT ( 'NONE',  ( -2.000000000000001776, 5.388445916248354013E-16, -4.400000000000000355 ) ) ;
#3581=B_SPLINE_CURVE_WITH_KNOTS ( 'NONE', 3,
 ( #9732, #12526, #6592, #1722 ),
 .UNSPECIFIED., .F., .F.,
 ( 4, 4 ),
 ( 0.000000000000000000, 0.001126652051248517921 ),
 .UNSPECIFIED. ) ;
#3587=VECTOR ( 'NONE', #17285, 1000.000000000000114 ) ;
#3588=CARTESIAN_POINT ( 'NONE',  ( 10.47794484381774538, 0.2987243419133224775, 5.700000000000001954 ) ) ;
#3598=( GEOMETRIC_REPRESENTATION_CONTEXT ( 3 ) GLOBAL_UNCERTAINTY_ASSIGNED_CONTEXT ( ( #5770 ) ) GLOBAL_UNIT_ASSIGNED_CONTEXT ( ( #675, #19164, #18876 ) ) REPRESENTATION_CONTEXT ( 'NONE', 'WORKASPACE' ) );
#3606=CARTESIAN_POINT ( 'NONE',  ( 11.81249999590322552, -5.700000000000005507, 0.9027913098498173694 ) ) ;
#3608=AXIS2_PLACEMENT_3D ( 'NONE', #5667, #7656, #2863 ) ;
#3613=CARTESIAN_POINT ( 'NONE',  ( 7.812499995903224637, 0.9027913098498568933, -5.700000000000000178 ) ) ;
#3617=CARTESIAN_POINT ( 'NONE',  ( 9.468749997951615427, -3.954556930911881985, 2.873153789725797491 ) ) ;
#3639=CARTESIAN_POINT ( 'NONE',  ( 8.312499995903225525, -3.814044456245443193, -4.235925505221191933 ) ) ;
#3644=ORIENTED_EDGE ( 'NONE', *, *, #5582, .F. ) ;
#3645=CARTESIAN_POINT ( 'NONE',  ( 6.843749997951615427, 4.233219804643871598, 2.444050593750020095 ) ) ;
#3646=CARTESIAN_POINT ( 'NONE',  ( 10.84374999795161543, 3.632567103900523620, 3.270778111535338262 ) ) ;
#3654=ORIENTED_EDGE ( 'NONE', *, *, #16122, .T. ) ;
#3661=ORIENTED_EDGE ( 'NONE', *, *, #16689, .F. ) ;
#3676=CARTESIAN_POINT ( 'NONE',  ( 8.812499995903225525, -3.143139765844555900, -4.840010801796527318 ) ) ;
#3685=DIRECTION ( 'NONE',  ( 0.000000000000000000, 0.000000000000000000, 1.000000000000000000 ) ) ;
#3694=CARTESIAN_POINT ( 'NONE',  ( 13.00000000000000533, -5.207209108562836697, 2.318398865532038666 ) ) ;
#3695=CARTESIAN_POINT ( 'NONE',  ( 8.343749997951611874, -4.942249507334558700, 0.2590123213420631454 ) ) ;
#3717=VERTEX_POINT ( 'NONE', #10038 ) ;
#3723=DIRECTION ( 'NONE',  ( 0.000000000000000000, 0.000000000000000000, -1.000000000000000000 ) ) ;
#3729=CARTESIAN_POINT ( 'NONE',  ( 6.843749997951615427, 4.233219804643887585, -2.444050593749990785 ) ) ;
#3735=ADVANCED_FACE ( 'NONE', ( #9013 ), #16627, .F. ) ;
#3744=EDGE_CURVE ( 'NONE', #16939, #7007, #4705, .T. ) ;
#3752=CARTESIAN_POINT ( 'NONE',  ( 6.000000000000005329, 0.000000000000000000, 0.000000000000000000 ) ) ;
#3756=EDGE_LOOP ( 'NONE', ( #13695, #6353, #8426, #17868, #16338, #14629 ) ) ;
#3768=EDGE_LOOP ( 'NONE', ( #11132, #10471, #6114, #17257 ) ) ;
#3776=CARTESIAN_POINT ( 'NONE',  ( 8.343749997951613651, -2.695436003842674122, -4.150607464521828938 ) ) ;
#3778=DIRECTION ( 'NONE',  ( -1.000000000000000000, 0.000000000000000000, 0.000000000000000000 ) ) ;
#3794=B_SPLINE_CURVE_WITH_KNOTS ( 'NONE', 3,
 ( #7782, #13894, #7149, #8383, #685, #11775, #6859, #8669, #17584, #17780 ),
 .UNSPECIFIED., .F., .F.,
 ( 4, 3, 3, 4 ),
 ( 0.000000000000000000, 0.0001875345074742634278, 0.0003808595644229697272, 0.0005744879655065562602 ),
 .UNSPECIFIED. ) ;
#3795=CARTESIAN_POINT ( 'NONE',  ( 9.343749997951615427, -4.780397808154247308, -1.280903732194487166 ) ) ;
#3812=EDGE_CURVE ( 'NONE', #3717, #10033, #8362, .T. ) ;
#3814=CARTESIAN_POINT ( 'NONE',  ( 13.96874999795161365, -3.499494075959791672, -3.499494075959840078 ) ) ;
#3822=CARTESIAN_POINT ( 'NONE',  ( 7.312499995903225525, 4.936344801571289409, 2.850000000000024070 ) ) ;
#3843=CARTESIAN_POINT ( 'NONE',  ( 9.343749997951615427, 1.280903732194421218, 4.780397808154266848 ) ) ;
#3854=ORIENTED_EDGE ( 'NONE', *, *, #11239, .T. ) ;
#3863=ORIENTED_EDGE ( 'NONE', *, *, #9847, .F. ) ;
#3869=CARTESIAN_POINT ( 'NONE',  ( 14.84374999795161543, 4.861323657744413218, -0.5109457054261112852 ) ) ;
#3870=CARTESIAN_POINT ( 'NONE',  ( 7.812499995903224637, -4.484949146646330931, -3.631840208645857437 ) ) ;
#3896=CARTESIAN_POINT ( 'NONE',  ( 8.843749997951615427, -2.873153789725853002, 3.954556930911842016 ) ) ;
#3902=AXIS2_PLACEMENT_3D ( 'NONE', #16015, #8418, #11512 ) ;
#3905=LINE ( 'NONE', #19016, #7737 ) ;
#3932=ORIENTED_EDGE ( 'NONE', *, *, #17857, .F. ) ;
#3946=ORIENTED_EDGE ( 'NONE', *, *, #4395, .F. ) ;
#3950=ADVANCED_FACE ( 'NONE', ( #106 ), #18668, .F. ) ;
#3958=CARTESIAN_POINT ( 'NONE',  ( 6.656249997951614539, 4.936344801571308061, -2.849999999999989431 ) ) ;
#3960=CARTESIAN_POINT ( 'NONE',  ( 0.000000000000000000, 0.000000000000000000, 5.700000000000001954 ) ) ;
#3966=PRESENTATION_STYLE_ASSIGNMENT (( #2363 ) ) ;
#3991=CYLINDRICAL_SURFACE ( 'NONE', #5207, 5.400000000000000355 ) ;
#4013=CARTESIAN_POINT ( 'NONE',  ( 11.31249999590322375, -4.235925505221111997, -3.814044456245531567 ) ) ;
#4041=FACE_OUTER_BOUND ( 'NONE', #1306, .T. ) ;
#4043=EDGE_CURVE ( 'NONE', #9272, #13507, #917, .T. ) ;
#4044=EDGE_CURVE ( 'NONE', #11866, #18865, #3065, .T. ) ;
#4048=CARTESIAN_POINT ( 'NONE',  ( 8.500000000000005329, 1.493657965219485018, 5.574407415329170057 ) ) ;
#4055=ORIENTED_EDGE ( 'NONE', *, *, #2952, .F. ) ;
#4056=CARTESIAN_POINT ( 'NONE',  ( 7.078124996927420476, -4.584782303107560963, -2.647025296875054057 ) ) ;
#4057=CARTESIAN_POINT ( 'NONE',  ( 7.312499995903225525, -4.936344801571327601, 2.849999999999954348 ) ) ;
#4065=EDGE_CURVE ( 'NONE', #18486, #4381, #15735, .T. ) ;
#4074=CARTESIAN_POINT ( 'NONE',  ( 7.343749997951615427, -3.846120219227900705, -3.114526743279308896 ) ) ;
#4083=CARTESIAN_POINT ( 'NONE',  ( 8.343749997951613651, -4.942249507334558700, 0.2590123213420630899 ) ) ;
#4089=LINE ( 'NONE', #13480, #12079 ) ;
#4118=EDGE_LOOP ( 'NONE', ( #6163, #19732, #11072, #4810, #13734 ) ) ;
#4122=ORIENTED_EDGE ( 'NONE', *, *, #8103, .T. ) ;
#4131=CARTESIAN_POINT ( 'NONE',  ( 12.92161831991541554, -3.713244971082748425, 3.181176262573032432 ) ) ;
#4138=CARTESIAN_POINT ( 'NONE',  ( 6.968749997951614539, 3.846120219227923798, 3.114526743279282694 ) ) ;
#4149=VERTEX_POINT ( 'NONE', #9775 ) ;
#4179=CARTESIAN_POINT ( 'NONE',  ( 12.34374999795161543, 1.773574444220725743, 4.620319390059829168 ) ) ;
#4190=CARTESIAN_POINT ( 'NONE',  ( 12.99999999999999467, 4.416988234087969367, 2.093740232017179181 ) ) ;
#4191=EDGE_CURVE ( 'NONE', #18200, #5529, #14946, .T. ) ;
#4193=ADVANCED_FACE ( 'NONE', ( #13256 ), #19342, .T. ) ;
#4197=CARTESIAN_POINT ( 'NONE',  ( 9.312499995903225525, 2.318398865532038666, 5.207209108562838473 ) ) ;
#4198=CARTESIAN_POINT ( 'NONE',  ( 10.81249999590322375, -4.840010801796461593, -3.143139765844656708 ) ) ;
#4207=CARTESIAN_POINT ( 'NONE',  ( 13.00000000000000533, -4.611396867937178179, -3.350375938067128967 ) ) ;
#4208=ORIENTED_EDGE ( 'NONE', *, *, #660, .T. ) ;
#4211=CARTESIAN_POINT ( 'NONE',  ( 9.968749997951615427, -4.409619785863921670, 2.246813503491803310 ) ) ;
#4219=AXIS2_PLACEMENT_3D ( 'NONE', #1497, #13397, #10703 ) ;
#4227=CARTESIAN_POINT ( 'NONE',  ( 13.00000000000000000, 4.125339889944109828, -2.622041954598519187 ) ) ;
#4258=CARTESIAN_POINT ( 'NONE',  ( 8.468749997951615427, -4.861323657744403448, -0.5109457054262123155 ) ) ;
#4265=CARTESIAN_POINT ( 'NONE',  ( 6.968749997951614539, 3.846120219227923798, 3.114526743279282694 ) ) ;
#4267=ORIENTED_EDGE ( 'NONE', *, *, #18874, .F. ) ;
#4290=CARTESIAN_POINT ( 'NONE',  ( 13.00000000000000178, 4.545788521379996006, 1.798195097859992098 ) ) ;
#4295=CARTESIAN_POINT ( 'NONE',  ( 10.31249999590322552, 0.5958122406255991210, 5.668774803599163192 ) ) ;
#4298=CARTESIAN_POINT ( 'NONE',  ( 12.73273607671833929, 3.906077990787180099, -2.967013497616978412 ) ) ;
#4299=CARTESIAN_POINT ( 'NONE',  ( 9.000000000000005329, 5.207209108562820710, 2.318398865532074193 ) ) ;
#4302=FACE_OUTER_BOUND ( 'NONE', #6234, .T. ) ;
#4311=CARTESIAN_POINT ( 'NONE',  ( 9.468749997951615427, 3.954556930911862000, -2.873153789725825469 ) ) ;
#4327=CARTESIAN_POINT ( 'NONE',  ( 12.34374999795161543, 1.773574444220725743, 4.620319390059829168 ) ) ;
#4340=CARTESIAN_POINT ( 'NONE',  ( 7.968749997951616315, -4.942249507334558700, 0.2590123213420631454 ) ) ;
#4341=CARTESIAN_POINT ( 'NONE',  ( 9.468749997951615427, 4.465502636338023912, 1.988169868018593300 ) ) ;
#4365=CARTESIAN_POINT ( 'NONE',  ( 13.50000000000000533, -5.574407415329169169, 1.493657965219485462 ) ) ;
#4372=ORIENTED_EDGE ( 'NONE', *, *, #14387, .T. ) ;
#4373=EDGE_CURVE ( 'NONE', #2730, #2350, #5794, .T. ) ;
#4376=CARTESIAN_POINT ( 'NONE',  ( 8.812499995903225525, 2.620002426024544029, -5.142044285764750811 ) ) ;
#4381=VERTEX_POINT ( 'NONE', #13842 ) ;
#4386=CARTESIAN_POINT ( 'NONE',  ( -2.000000000000001776, 3.218695387886217230, -3.000000000000000000 ) ) ;
#4395=EDGE_CURVE ( 'NONE', #4149, #6896, #5109, .T. ) ;
#4396=CARTESIAN_POINT ( 'NONE',  ( 6.968749997951614539, -3.846120219227900705, -3.114526743279308896 ) ) ;
#4397=CARTESIAN_POINT ( 'NONE',  ( 8.500000000000005329, 5.574407415329157622, 1.493657965219523875 ) ) ;
#4403=CARTESIAN_POINT ( 'NONE',  ( 14.00000000000000533, -3.350375938067065906, -4.611396867937224364 ) ) ;
#4404=EDGE_LOOP ( 'NONE', ( #8244, #6068, #17246, #145 ) ) ;
#4410=DIRECTION ( 'NONE',  ( 0.000000000000000000, 6.982962677686267499E-15, -1.000000000000000000 ) ) ;
#4418=EDGE_CURVE ( 'NONE', #6896, #10630, #19163, .T. ) ;
#4419=DIRECTION ( 'NONE',  ( 0.000000000000000000, 0.000000000000000000, 1.000000000000000000 ) ) ;
#4437=CARTESIAN_POINT ( 'NONE',  ( 13.00000000000000533, 4.560365019702147471, 2.978280878416429633 ) ) ;
#4442=DIRECTION ( 'NONE',  ( 0.000000000000000000, 0.000000000000000000, 1.000000000000000000 ) ) ;
#4453=CARTESIAN_POINT ( 'NONE',  ( 9.468749997951615427, -4.465502636338009701, -1.988169868018624609 ) ) ;
#4467=CARTESIAN_POINT ( 'NONE',  ( 6.000593838912648081, -0.002144393866035136480, 5.699999596629369059 ) ) ;
#4473=CARTESIAN_POINT ( 'NONE',  ( 6.234374998975811266, -3.696815770993907903E-14, 5.294050593750000644 ) ) ;
#4479=DIRECTION ( 'NONE',  ( 1.000000000000000000, 0.000000000000000000, 0.000000000000000000 ) ) ;
#4486=VECTOR ( 'NONE', #4479, 1000.000000000000000 ) ;
#4487=EDGE_LOOP ( 'NONE', ( #16822, #9810, #13995, #9536 ) ) ;
#4488=CARTESIAN_POINT ( 'NONE',  ( 12.31249999590322552, -2.850000000000023626, 4.936344801571289409 ) ) ;
#4491=CARTESIAN_POINT ( 'NONE',  ( 10.46874999795161720, 1.016293382781477961, -4.781284448697179279 ) ) ;
#4500=CARTESIAN_POINT ( 'NONE',  ( 7.843749997951614539, 1.510506337161861445, -4.648860486681953397 ) ) ;
#4515=CARTESIAN_POINT ( 'NONE',  ( 13.81249999590322552, 0.3020334839682480288, 5.763142191869157216 ) ) ;
#4517=EDGE_LOOP ( 'NONE', ( #13105, #6804 ) ) ;
#4538=VERTEX_POINT ( 'NONE', #3822 ) ;
#4558=CARTESIAN_POINT ( 'NONE',  ( 11.84374999795161365, 4.888101187500000222, -2.993098736590125853E-16 ) ) ;
#4568=EDGE_CURVE ( 'NONE', #720, #18915, #16032, .T. ) ;
#4571=CARTESIAN_POINT ( 'NONE',  ( 10.31249999590322552, 4.611396867937201272, -3.350375938067097437 ) ) ;
#4590=CARTESIAN_POINT ( 'NONE',  ( 10.50000000000000711, 2.068159791354259092, -5.387740456496206143 ) ) ;
#4595=AXIS2_PLACEMENT_3D ( 'NONE', #18890, #6865, #8390 ) ;
#4600=CARTESIAN_POINT ( 'NONE',  ( 2.999999999999998224, 2.487173708821167839, -2.318181818181817899 ) ) ;
#4610=DIRECTION ( 'NONE',  ( 1.000000000000000000, 0.000000000000000000, 0.000000000000000000 ) ) ;
#4615=CARTESIAN_POINT ( 'NONE',  ( 7.343749997951615427, -0.7741991708319229115, 4.888101187499994893 ) ) ;
#4634=CARTESIAN_POINT ( 'NONE',  ( 6.968749997951614539, 4.620319390059829168, -1.773574444220725077 ) ) ;
#4656=DIRECTION ( 'NONE',  ( -1.000000000000000000, 0.000000000000000000, 0.000000000000000000 ) ) ;
#4657=DIRECTION ( 'NONE',  ( 0.000000000000000000, 0.000000000000000000, 1.000000000000000000 ) ) ;
#4666=ORIENTED_EDGE ( 'NONE', *, *, #19645, .F. ) ;
#4671=ADVANCED_FACE ( 'NONE', ( #4 ), #8917, .T. ) ;
#4686=FACE_OUTER_BOUND ( 'NONE', #5949, .T. ) ;
#4689=EDGE_LOOP ( 'NONE', ( #19116, #11764, #16082, #7648 ) ) ;
#4693=CIRCLE ( 'NONE', #211, 5.700000000000001954 ) ;
#4697=ORIENTED_EDGE ( 'NONE', *, *, #6366, .F. ) ;
#4698=CARTESIAN_POINT ( 'NONE',  ( 7.000000000000005329, 1.761396867937200517, -5.421022142882375938 ) ) ;
#4703=CARTESIAN_POINT ( 'NONE',  ( 12.96874999795161543, -4.150607464521812062, 2.695436003842704764 ) ) ;
#4704=CARTESIAN_POINT ( 'NONE',  ( 12.50000000000000533, 0.3020334839682475847, 5.763142191869157216 ) ) ;
#4705=CIRCLE ( 'NONE', #8853, 5.700000000000001954 ) ;
#4722=CARTESIAN_POINT ( 'NONE',  ( 9.468749997951615427, 3.954556930911862000, -2.873153789725825469 ) ) ;
#4735=CARTESIAN_POINT ( 'NONE',  ( 2.999999999999998224, 0.000000000000000000, 0.000000000000000000 ) ) ;
#4739=DIRECTION ( 'NONE',  ( -1.000000000000000000, -0.000000000000000000, -0.000000000000000000 ) ) ;
#4743=CARTESIAN_POINT ( 'NONE',  ( 14.34374999795161365, 4.780397808154273065, -1.280903732194386802 ) ) ;
#4749=CARTESIAN_POINT ( 'NONE',  ( 6.000000000000005329, 0.000000000000000000, 0.000000000000000000 ) ) ;
#4787=CARTESIAN_POINT ( 'NONE',  ( 8.500000000000007105, -1.493657965219446382, -5.574407415329178939 ) ) ;
#4794=VERTEX_POINT ( 'NONE', #210 ) ;
#4802=CARTESIAN_POINT ( 'NONE',  ( 7.468749997951615427, 4.781284448697194378, -1.016293382781411125 ) ) ;
#4803=ADVANCED_FACE ( 'NONE', ( #17309 ), #12617, .F. ) ;
#4810=ORIENTED_EDGE ( 'NONE', *, *, #5582, .T. ) ;
#4823=ORIENTED_EDGE ( 'NONE', *, *, #10042, .F. ) ;
#4844=FACE_OUTER_BOUND ( 'NONE', #2817, .T. ) ;
#4882=EDGE_LOOP ( 'NONE', ( #16886, #6164, #8380, #7752, #5234 ) ) ;
#4889=EDGE_CURVE ( 'NONE', #18915, #16413, #808, .T. ) ;
#4895=ORIENTED_EDGE ( 'NONE', *, *, #14470, .T. ) ;
#4916=CARTESIAN_POINT ( 'NONE',  ( 9.332722423957255486, 2.725425358843983450E-16, 5.700000000000002842 ) ) ;
#4934=DIRECTION ( 'NONE',  ( 0.000000000000000000, 0.000000000000000000, -1.000000000000000000 ) ) ;
#4937=AXIS2_PLACEMENT_3D ( 'NONE', #6422, #11639, #19048 ) ;
#4940=ORIENTED_EDGE ( 'NONE', *, *, #14097, .F. ) ;
#4941=EDGE_CURVE ( 'NONE', #2350, #13507, #8675, .T. ) ;
#4953=CARTESIAN_POINT ( 'NONE',  ( 9.332722423957255486, 2.725425358843983450E-16, 5.700000000000002842 ) ) ;
#4954=CARTESIAN_POINT ( 'NONE',  ( 13.34374999795161365, 0.2590123213420971182, 4.942249507334556924 ) ) ;
#4958=CARTESIAN_POINT ( 'NONE',  ( 13.00000000000000000, -1.727010089215899713, -5.432074755721473025 ) ) ;
#4972=ORIENTED_EDGE ( 'NONE', *, *, #713, .F. ) ;
#4978=ORIENTED_EDGE ( 'NONE', *, *, #4941, .F. ) ;
#4990=CARTESIAN_POINT ( 'NONE',  ( 7.500000000000005329, 2.620002426024544029, -5.142044285764750811 ) ) ;
#4995=CARTESIAN_POINT ( 'NONE',  ( 8.312499995903225525, 5.575441324182696334, -1.185096637661215535 ) ) ;
#4998=CARTESIAN_POINT ( 'NONE',  ( 6.468749997951615427, 4.233219804643871598, 2.444050593750020095 ) ) ;
#5001=( BOUNDED_CURVE ( )  B_SPLINE_CURVE ( 2, ( #8427, #14535, #6899, #13028, #918, #6996, #17720, #19213, #4013, #10124, #13610, #1507, #1305 ),
 .UNSPECIFIED., .F., .F. ) 
 B_SPLINE_CURVE_WITH_KNOTS ( ( 3, 2, 2, 2, 2, 2, 3 ),
 ( 0.000000000000000000, 0.05000000000000000278, 0.1000000000000000056, 0.1499999999999999944, 0.2000000000000000111, 0.2500000000000000000, 0.2843253191101273170 ),
 .UNSPECIFIED. ) 
 CURVE ( )  GEOMETRIC_REPRESENTATION_ITEM ( )  RATIONAL_B_SPLINE_CURVE ( ( 1.000000000000000000, 0.9876883405951377704, 1.000000000000000000, 0.9876883405951377704, 1.000000000000000000, 0.9876883405951377704, 1.000000000000000000, 0.9876883405951377704, 1.000000000000000000, 0.9876883405951377704, 1.000000000000000000, 0.9915479672430580482, 0.9947006833465674713 ) ) 
 REPRESENTATION_ITEM ( '' )  );
#5006=CARTESIAN_POINT ( 'NONE',  ( 12.46874999795161543, -4.648860486681943627, -1.510506337161893642 ) ) ;
#5009=EDGE_CURVE ( 'NONE', #2569, #6283, #10302, .T. ) ;
#5021=VERTEX_POINT ( 'NONE', #14996 ) ;
#5022=CARTESIAN_POINT ( 'NONE',  ( -2.000000000000001776, 3.218695387886217674, -3.000000000000000000 ) ) ;
#5038=CARTESIAN_POINT ( 'NONE',  ( 10.50000000000000533, -3.631840208645763735, -4.484949146646406426 ) ) ;
#5052=CARTESIAN_POINT ( 'NONE',  ( 13.00000000000000178, -0.7793280607714923036, -4.825575716215948496 ) ) ;
#5058=CARTESIAN_POINT ( 'NONE',  ( 2.999999999999998224, 3.218695387886217230, 3.000000000000000000 ) ) ;
#5065=ORIENTED_EDGE ( 'NONE', *, *, #19459, .T. ) ;
#5074=DIRECTION ( 'NONE',  ( 0.000000000000000000, 0.000000000000000000, 1.000000000000000000 ) ) ;
#5079=ADVANCED_FACE ( 'NONE', ( #2554 ), #14682, .F. ) ;
#5102=CARTESIAN_POINT ( 'NONE',  ( 11.00000000000000711, -2.850000000000023626, 4.936344801571289409 ) ) ;
#5107=CARTESIAN_POINT ( 'NONE',  ( 9.968749997951617203, -4.409619785863921670, 2.246813503491803310 ) ) ;
#5109=( BOUNDED_CURVE ( )  B_SPLINE_CURVE ( 2, ( #18344, #4634, #6218, #16645, #10646, #12345, #4341, #1538, #15349, #13740, #15445, #1631, #3028, #2926, #1736 ),
 .UNSPECIFIED., .F., .F. ) 
 B_SPLINE_CURVE_WITH_KNOTS ( ( 3, 2, 2, 2, 2, 2, 2, 3 ),
 ( 0.000000000000000000, 0.05000000000000000971, 0.1000000000000000194, 0.1499999999999999944, 0.2000000000000000389, 0.2500000000000000000, 0.2999999999999999889, 0.3265529187307102399 ),
 .UNSPECIFIED. ) 
 CURVE ( )  GEOMETRIC_REPRESENTATION_ITEM ( )  RATIONAL_B_SPLINE_CURVE ( ( 1.000000000000000000, 0.9876883405951377704, 1.000000000000000000, 0.9876883405951377704, 1.000000000000000000, 0.9876883405951377704, 1.000000000000000000, 0.9876883405951377704, 1.000000000000000000, 0.9876883405951377704, 1.000000000000000000, 0.9876883405951377704, 1.000000000000000000, 0.9934617901676501273, 0.9938679225082089896 ) ) 
 REPRESENTATION_ITEM ( '' )  );
#5132=CARTESIAN_POINT ( 'NONE',  ( 10.34374999795161543, -0.2590123213421313686, 4.942249507334556036 ) ) ;
#5137=CARTESIAN_POINT ( 'NONE',  ( 10.34374999795161543, -0.2590123213421313686, 4.942249507334556036 ) ) ;
#5138=DIRECTION ( 'NONE',  ( -1.000000000000000000, 0.000000000000000000, 0.000000000000000000 ) ) ;
#5140=VERTEX_POINT ( 'NONE', #781 ) ;
#5145=ORIENTED_EDGE ( 'NONE', *, *, #5009, .F. ) ;
#5149=AXIS2_PLACEMENT_3D ( 'NONE', #15420, #18418, #1903 ) ;
#5169=LINE ( 'NONE', #11185, #3587 ) ;
#5179=LINE ( 'NONE', #11298, #18657 ) ;
#5188=CARTESIAN_POINT ( 'NONE',  ( -0.000000000000000000, 0.000000000000000000, 0.000000000000000000 ) ) ;
#5192=CARTESIAN_POINT ( 'NONE',  ( 7.343749997951615427, -4.620319390059841602, 1.773574444220693103 ) ) ;
#5197=CARTESIAN_POINT ( 'NONE',  ( 7.312499995903225525, -3.980288726281172656E-14, 5.700000000000001066 ) ) ;
#5200=VECTOR ( 'NONE', #8561, 1000.000000000000000 ) ;
#5207=AXIS2_PLACEMENT_3D ( 'NONE', #14894, #1184, #19001 ) ;
#5209=CARTESIAN_POINT ( 'NONE',  ( 13.00000000000000533, -5.207209108562836697, 2.318398865532038666 ) ) ;
#5210=ORIENTED_EDGE ( 'NONE', *, *, #1555, .F. ) ;
#5221=PRODUCT ( 'CLUTCH CONE', 'CLUTCH CONE', '', ( #9463 ) ) ;
#5234=ORIENTED_EDGE ( 'NONE', *, *, #6140, .F. ) ;
#5239=ORIENTED_EDGE ( 'NONE', *, *, #2480, .T. ) ;
#5245=ORIENTED_EDGE ( 'NONE', *, *, #7855, .T. ) ;
#5248=CARTESIAN_POINT ( 'NONE',  ( 9.332722423957255486, 2.725425358843983450E-16, 5.700000000000002842 ) ) ;
#5250=ORIENTED_EDGE ( 'NONE', *, *, #18777, .T. ) ;
#5278=LINE ( 'NONE', #17489, #18385 ) ;
#5281=CARTESIAN_POINT ( 'NONE',  ( 12.00000000000000533, 5.421022142882376826, 1.761396867937200073 ) ) ;
#5296=CARTESIAN_POINT ( 'NONE',  ( 12.34374999795161543, -1.773574444220693325, -4.620319390059841602 ) ) ;
#5302=CARTESIAN_POINT ( 'NONE',  ( 7.812499995903224637, -0.9027913098498965283, 5.699999999999994849 ) ) ;
#5327=VERTEX_POINT ( 'NONE', #2857 ) ;
#5336=CARTESIAN_POINT ( 'NONE',  ( 13.00000000000000178, -0.5876048313370498821, -4.852654302691288279 ) ) ;
#5339=ORIENTED_EDGE ( 'NONE', *, *, #8678, .T. ) ;
#5341=CYLINDRICAL_SURFACE ( 'NONE', #8674, 4.400000000000000355 ) ;
#5342=ORIENTED_EDGE ( 'NONE', *, *, #1443, .T. ) ;
#5345=DIRECTION ( 'NONE',  ( 0.000000000000000000, 0.000000000000000000, 1.000000000000000000 ) ) ;
#5368=VECTOR ( 'NONE', #14611, 1000.000000000000114 ) ;
#5370=CARTESIAN_POINT ( 'NONE',  ( 13.84374999795161543, 4.465502636338051445, -1.988169868018530906 ) ) ;
#5377=CARTESIAN_POINT ( 'NONE',  ( 11.34374999795161543, -3.114526743279228072, -3.846120219227966430 ) ) ;
#5396=CARTESIAN_POINT ( 'NONE',  ( 11.34374999795161543, -4.888101187500005551, 0.7741991708318548548 ) ) ;
#5423=DIRECTION ( 'NONE',  ( -1.000000000000000000, 0.000000000000000000, 0.000000000000000000 ) ) ;
#5442=CARTESIAN_POINT ( 'NONE',  ( 8.000000000000005329, 2.318398865532038666, 5.207209108562838473 ) ) ;
#5450=DIRECTION ( 'NONE',  ( 1.000000000000000000, 0.000000000000000000, 0.000000000000000000 ) ) ;
#5452=B_SPLINE_CURVE_WITH_KNOTS ( 'NONE', 3,
 ( #12987, #13277, #11675, #15985, #10090, #16282, #9798, #878, #6764, #11387 ),
 .UNSPECIFIED., .F., .F.,
 ( 4, 3, 3, 4 ),
 ( 0.000000000000000000, 0.0001875345074742618286, 0.0003808595644229699983, 0.0005744879655065563686 ),
 .UNSPECIFIED. ) ;
#5462=VERTEX_POINT ( 'NONE', #17143 ) ;
#5464=CARTESIAN_POINT ( 'NONE',  ( 7.312499995903225525, 4.936344801571308061, -2.849999999999989431 ) ) ;
#5472=CYLINDRICAL_SURFACE ( 'NONE', #4595, 4.400000000000000355 ) ;
#5473=CARTESIAN_POINT ( 'NONE',  ( 9.343749997951615427, -4.780397808154247308, -1.280903732194487166 ) ) ;
#5474=CARTESIAN_POINT ( 'NONE',  ( 9.812499995903225525, 1.493657965219485018, 5.574407415329170057 ) ) ;
#5486=CARTESIAN_POINT ( 'NONE',  ( 12.81249999590322552, -5.699999999999994849, -0.9027913098498961952 ) ) ;
#5491=ORIENTED_EDGE ( 'NONE', *, *, #19459, .F. ) ;
#5492=CARTESIAN_POINT ( 'NONE',  ( 2.999999999999998224, 0.000000000000000000, 0.000000000000000000 ) ) ;
#5503=AXIS2_PLACEMENT_3D ( 'NONE', #12778, #2164, #11277 ) ;
#5504=CARTESIAN_POINT ( 'NONE',  ( 13.00000000000000533, -0.5958122406256377568, 5.668774803599156975 ) ) ;
#5520=EDGE_CURVE ( 'NONE', #18200, #3546, #15869, .T. ) ;
#5521=CARTESIAN_POINT ( 'NONE',  ( 6.656249997951614539, 4.233219804643871598, 2.444050593750020095 ) ) ;
#5528=CARTESIAN_POINT ( 'NONE',  ( 6.468749997951615427, 0.000000000000000000, -4.888101187500000222 ) ) ;
#5529=VERTEX_POINT ( 'NONE', #10233 ) ;
#5533=LINE ( 'NONE', #2627, #2264 ) ;
#5547=LINE ( 'NONE', #4056, #14039 ) ;
#5548=CARTESIAN_POINT ( 'NONE',  ( 6.500000000000005329, -0.9027913098498966393, 5.699999999999994849 ) ) ;
#5551=MECHANICAL_DESIGN_GEOMETRIC_PRESENTATION_REPRESENTATION('',(#16753),#17699);
#5554=VERTEX_POINT ( 'NONE', #19318 ) ;
#5580=DIRECTION ( 'NONE',  ( 0.000000000000000000, -0.4999999999999978906, -0.8660254037844399289 ) ) ;
#5582=EDGE_CURVE ( 'NONE', #6183, #10033, #14994, .T. ) ;
#5587=CARTESIAN_POINT ( 'NONE',  ( 14.34374999795161365, -4.780397808154265960, 1.280903732194421663 ) ) ;
#5589=AXIS2_PLACEMENT_3D ( 'NONE', #3752, #9875, #5345 ) ;
#5597=CARTESIAN_POINT ( 'NONE',  ( 11.00000000000000711, -5.700000000000001066, -3.945386292505473391E-14 ) ) ;
#5598=EDGE_LOOP ( 'NONE', ( #16045, #15744, #2442, #18269 ) ) ;
#5610=CARTESIAN_POINT ( 'NONE',  ( 11.81249999590322552, -2.068159791354220900, 5.387740456496221242 ) ) ;
#5618=CARTESIAN_POINT ( 'NONE',  ( 13.00000000000000178, -3.789407127742538517, 3.087705756618167374 ) ) ;
#5635=( BOUNDED_SURFACE ( )  B_SPLINE_SURFACE ( 1, 2, ( 
 ( #10791, #13893, #186, #6269, #12396, #18487, #16091, #18782, #12687, #6660, #17486, #2371, #8178, #1974, #5370, #14184, #3869 ),
 ( #12986, #6858, #15984, #2274, #2174, #11386, #12886, #18982, #8381, #17189, #9797, #9991, #485, #3573, #9589, #8485, #14496 ) ),
 .UNSPECIFIED., .F., .F., .F. ) 
 B_SPLINE_SURFACE_WITH_KNOTS ( ( 2, 2 ),
 ( 3, 2, 2, 2, 2, 2, 2, 2, 3 ),
 ( 0.000000000000000000, 1.000000000000000000 ),
 ( 0.000000000000000000, 0.05000000000000000278, 0.1000000000000000056, 0.1499999999999999944, 0.2000000000000000111, 0.2500000000000000000, 0.2999999999999999889, 0.3499999999999999778, 0.4000000000000000222 ),
 .UNSPECIFIED. ) 
 GEOMETRIC_REPRESENTATION_ITEM ( )  RATIONAL_B_SPLINE_SURFACE ( (
 ( 1.000000000000000000, 0.9876883405951377704, 1.000000000000000000, 0.9876883405951377704, 1.000000000000000000, 0.9876883405951377704, 1.000000000000000000, 0.9876883405951377704, 1.000000000000000000, 0.9876883405951377704, 1.000000000000000000, 0.9876883405951377704, 1.000000000000000000, 0.9876883405951377704, 1.000000000000000000, 0.9876883405951377704, 1.000000000000000000),
 ( 1.000000000000000000, 0.9876883405951377704, 1.000000000000000000, 0.9876883405951377704, 1.000000000000000000, 0.9876883405951377704, 1.000000000000000000, 0.9876883405951377704, 1.000000000000000000, 0.9876883405951377704, 1.000000000000000000, 0.9876883405951377704, 1.000000000000000000, 0.9876883405951377704, 1.000000000000000000, 0.9876883405951377704, 1.000000000000000000) ) ) 
 REPRESENTATION_ITEM ( '' )  SURFACE ( )  );
#5655=CARTESIAN_POINT ( 'NONE',  ( 8.468749997951615427, 1.988169868018562436, 4.465502636338039011 ) ) ;
#5661=CARTESIAN_POINT ( 'NONE',  ( 9.812499995903225525, -1.493657965219446160, -5.574407415329178939 ) ) ;
#5667=CARTESIAN_POINT ( 'NONE',  ( 6.234374998975811266, -4.584782303107560963, -2.647025296875054057 ) ) ;
#5668=CARTESIAN_POINT ( 'NONE',  ( 11.34374999795161543, 4.888101187500000222, -0.7741991708318890497 ) ) ;
#5684=FACE_OUTER_BOUND ( 'NONE', #19612, .T. ) ;
#5691=CARTESIAN_POINT ( 'NONE',  ( 8.968749997951611874, 3.499494075959816541, -3.499494075959816541 ) ) ;
#5694=CARTESIAN_POINT ( 'NONE',  ( 9.000000000000005329, -4.611396867937225252, 3.350375938067065462 ) ) ;
#5716=EDGE_CURVE ( 'NONE', #14637, #9343, #19365, .T. ) ;
#5719=ORIENTED_EDGE ( 'NONE', *, *, #11368, .F. ) ;
#5726=CARTESIAN_POINT ( 'NONE',  ( 12.96874999795161543, -0.2590123213420631454, -4.942249507334558700 ) ) ;
#5763=CARTESIAN_POINT ( 'NONE',  ( 12.92161831991541554, 0.8983569717629179552, 4.806352606718987452 ) ) ;
#5770=UNCERTAINTY_MEASURE_WITH_UNIT (LENGTH_MEASURE( 1.000000000000000082E-05 ), #675, 'distance_accuracy_value', 'NONE');
#5780=CARTESIAN_POINT ( 'NONE',  ( 9.843749997951615427, 0.5109457054261445919, 4.861323657744411442 ) ) ;
#5782=CARTESIAN_POINT ( 'NONE',  ( 8.812499995903225525, -5.763142191869158992, 0.3020334839682081163 ) ) ;
#5783=CARTESIAN_POINT ( 'NONE',  ( 11.96874999795161365, 3.114526743279308896, -3.846120219227901149 ) ) ;
#5790=DIRECTION ( 'NONE',  ( 1.000000000000000000, 0.000000000000000000, 0.000000000000000000 ) ) ;
#5794=B_SPLINE_CURVE_WITH_KNOTS ( 'NONE', 3,
 ( #18248, #4437, #2827, #6024 ),
 .UNSPECIFIED., .F., .F.,
 ( 4, 4 ),
 ( 0.000000000000000000, 0.001125480700308659687 ),
 .UNSPECIFIED. ) ;
#5796=CARTESIAN_POINT ( 'NONE',  ( 8.843749997951615427, 2.873153789725825469, -3.954556930911862000 ) ) ;
#5798=CARTESIAN_POINT ( 'NONE',  ( 13.00000000000000000, -4.333424887442987483, -2.261628166637620119 ) ) ;
#5803=DIRECTION ( 'NONE',  ( 0.000000000000000000, 0.000000000000000000, 1.000000000000000000 ) ) ;
#5814=CARTESIAN_POINT ( 'NONE',  ( 12.31249999590322552, 2.849999999999989875, 4.936344801571308061 ) ) ;
#5830=CARTESIAN_POINT ( 'NONE',  ( 12.99999999999999467, 0.4594918047638986702, 4.866883308198427294 ) ) ;
#5853=CARTESIAN_POINT ( 'NONE',  ( 8.968749997951611874, 1.280903732194421218, 4.780397808154266848 ) ) ;
#5863=B_SPLINE_CURVE_WITH_KNOTS ( 'NONE', 3,
 ( #15757, #8144, #15461, #7840 ),
 .UNSPECIFIED., .F., .F.,
 ( 4, 4 ),
 ( 0.000000000000000000, 0.001125480700308659687 ),
 .UNSPECIFIED. ) ;
#5877=PLANE ( 'NONE',  #16058 ) ;
#5889=CARTESIAN_POINT ( 'NONE',  ( 10.00000000000000533, 4.235925505221138643, 3.814044456245502701 ) ) ;
#5896=CARTESIAN_POINT ( 'NONE',  ( 9.500000000000003553, -5.142044285764769462, 2.620002426024508502 ) ) ;
#5901=CARTESIAN_POINT ( 'NONE',  ( 10.96874999795161720, -4.888101187500005551, 0.7741991708318548548 ) ) ;
#5913=EDGE_LOOP ( 'NONE', ( #17559, #10881, #5961, #16495, #8029, #6339, #12480, #3054, #17833, #18878 ) ) ;
#5915=CARTESIAN_POINT ( 'NONE',  ( 9.968749997951615427, 4.409619785863906571, -2.246813503491833508 ) ) ;
#5916=EDGE_LOOP ( 'NONE', ( #12073, #5975, #18753, #8777 ) ) ;
#5921=ORIENTED_EDGE ( 'NONE', *, *, #17482, .F. ) ;
#5926=CARTESIAN_POINT ( 'NONE',  ( 6.000000000000005329, -4.936344801571327601, 2.849999999999954348 ) ) ;
#5943=ORIENTED_EDGE ( 'NONE', *, *, #17482, .T. ) ;
#5947=PLANE ( 'NONE',  #9584 ) ;
#5949=EDGE_LOOP ( 'NONE', ( #17232, #381, #9889, #10604 ) ) ;
#5950=CARTESIAN_POINT ( 'NONE',  ( 6.000000000000005329, 0.000000000000000000, 0.000000000000000000 ) ) ;
#5961=ORIENTED_EDGE ( 'NONE', *, *, #12376, .T. ) ;
#5972=VECTOR ( 'NONE', #10034, 1000.000000000000000 ) ;
#5973=CARTESIAN_POINT ( 'NONE',  ( 13.00000000000000000, 4.362347728716210682, 2.206210144330583933 ) ) ;
#5975=ORIENTED_EDGE ( 'NONE', *, *, #16350, .T. ) ;
#5978=ORIENTED_EDGE ( 'NONE', *, *, #4941, .T. ) ;
#5979=CARTESIAN_POINT ( 'NONE',  ( 11.84374999795161365, -2.444050593750019651, 4.233219804643871598 ) ) ;
#5985=EDGE_CURVE ( 'NONE', #2730, #12192, #4693, .T. ) ;
#5995=CARTESIAN_POINT ( 'NONE',  ( 8.968749997951613651, -3.499494075959840966, 3.499494075959792116 ) ) ;
#5996=CARTESIAN_POINT ( 'NONE',  ( 13.96874999795161365, 3.499494075959816541, 3.499494075959815653 ) ) ;
#5999=ORIENTED_EDGE ( 'NONE', *, *, #14097, .T. ) ;
#6002=CARTESIAN_POINT ( 'NONE',  ( -2.000000000000001776, 0.000000000000000000, 0.000000000000000000 ) ) ;
#6011=CARTESIAN_POINT ( 'NONE',  ( 14.31249999590322552, -0.5958122406256373127, 5.668774803599156975 ) ) ;
#6023=CARTESIAN_POINT ( 'NONE',  ( 6.468749997951615427, -4.233219804643904460, 2.444050593749960587 ) ) ;
#6024=CARTESIAN_POINT ( 'NONE',  ( 13.00000000000000000, 4.333424887443004359, 2.261628166637590365 ) ) ;
#6036=CARTESIAN_POINT ( 'NONE',  ( 2.999999999999998224, -3.950217066951263956, -3.681818181818183877 ) ) ;
#6048=CARTESIAN_POINT ( 'NONE',  ( 10.34374999795161543, 4.409619785863906571, -2.246813503491833508 ) ) ;
#6050=ADVANCED_FACE ( 'NONE', ( #11506 ), #710, .T. ) ;
#6068=ORIENTED_EDGE ( 'NONE', *, *, #18706, .T. ) ;
#6081=CARTESIAN_POINT ( 'NONE',  ( 7.843749997951614539, -4.781284448697200595, 1.016293382781377819 ) ) ;
#6093=CARTESIAN_POINT ( 'NONE',  ( 12.46874999795161543, -4.648860486681943627, -1.510506337161893642 ) ) ;
#6100=CARTESIAN_POINT ( 'NONE',  ( 9.843749997951615427, -3.954556930911881985, 2.873153789725797491 ) ) ;
#6108=DIRECTION ( 'NONE',  ( 0.000000000000000000, 0.000000000000000000, 1.000000000000000000 ) ) ;
#6114=ORIENTED_EDGE ( 'NONE', *, *, #18465, .T. ) ;
#6116=ORIENTED_EDGE ( 'NONE', *, *, #1443, .F. ) ;
#6128=DIRECTION ( 'NONE',  ( 0.000000000000000000, 0.000000000000000000, 1.000000000000000000 ) ) ;
#6131=LINE ( 'NONE', #10748, #10009 ) ;
#6136=CARTESIAN_POINT ( 'NONE',  ( 6.000000000000005329, -4.936344801571327601, 2.849999999999954348 ) ) ;
#6140=EDGE_CURVE ( 'NONE', #5140, #15581, #2075, .T. ) ;
#6149=CARTESIAN_POINT ( 'NONE',  ( 12.84374999795161543, 4.648860486681953397, 1.510506337161861223 ) ) ;
#6163=ORIENTED_EDGE ( 'NONE', *, *, #1499, .F. ) ;
#6164=ORIENTED_EDGE ( 'NONE', *, *, #6233, .F. ) ;
#6166=PRESENTATION_STYLE_ASSIGNMENT (( #16492 ) ) ;
#6168=EDGE_LOOP ( 'NONE', ( #8836, #19763, #1398, #2756 ) ) ;
#6183=VERTEX_POINT ( 'NONE', #11998 ) ;
#6184=CARTESIAN_POINT ( 'NONE',  ( 14.00000000000000533, 3.350375938067097881, 4.611396867937200383 ) ) ;
#6191=CARTESIAN_POINT ( 'NONE',  ( 14.84374999795161543, -4.861323657744410554, 0.5109457054261454800 ) ) ;
#6201=EDGE_LOOP ( 'NONE', ( #11466, #3863, #19502, #12108 ) ) ;
#6218=CARTESIAN_POINT ( 'NONE',  ( 7.468749997951615427, 4.781284448697194378, -1.016293382781411125 ) ) ;
#6230=DIRECTION ( 'NONE',  ( 1.000000000000000000, 0.000000000000000000, 0.000000000000000000 ) ) ;
#6233=EDGE_CURVE ( 'NONE', #4149, #11016, #13994, .T. ) ;
#6234=EDGE_LOOP ( 'NONE', ( #11776, #7666, #2306, #3265 ) ) ;
#6252=CARTESIAN_POINT ( 'NONE',  ( 8.343749997951613651, 2.695436003842704764, 4.150607464521811174 ) ) ;
#6269=CARTESIAN_POINT ( 'NONE',  ( 8.343749997951611874, -2.695436003842674566, -4.150607464521828938 ) ) ;
#6271=( BOUNDED_SURFACE ( )  B_SPLINE_SURFACE ( 1, 2, ( 
 ( #8141, #10853, #3639, #11048, #17154, #6622, #448, #2038, #12654, #1747, #16959, #9556, #6524, #13952, #1937, #9761, #13854 ),
 ( #11151, #17351, #3538, #3444, #243, #1645, #10952, #147, #17058, #18846, #554, #17248, #12452, #12358, #7935, #4743, #9656 ) ),
 .UNSPECIFIED., .F., .F., .F. ) 
 B_SPLINE_SURFACE_WITH_KNOTS ( ( 2, 2 ),
 ( 3, 2, 2, 2, 2, 2, 2, 2, 3 ),
 ( 0.000000000000000000, 1.000000000000000000 ),
 ( 0.000000000000000000, 0.05000000000000000278, 0.1000000000000000056, 0.1499999999999999944, 0.2000000000000000111, 0.2500000000000000000, 0.2999999999999999889, 0.3499999999999999778, 0.4000000000000000222 ),
 .UNSPECIFIED. ) 
 GEOMETRIC_REPRESENTATION_ITEM ( )  RATIONAL_B_SPLINE_SURFACE ( (
 ( 1.000000000000000000, 0.9876883405951377704, 1.000000000000000000, 0.9876883405951377704, 1.000000000000000000, 0.9876883405951377704, 1.000000000000000000, 0.9876883405951377704, 1.000000000000000000, 0.9876883405951377704, 1.000000000000000000, 0.9876883405951377704, 1.000000000000000000, 0.9876883405951377704, 1.000000000000000000, 0.9876883405951377704, 1.000000000000000000),
 ( 1.000000000000000000, 0.9876883405951377704, 1.000000000000000000, 0.9876883405951377704, 1.000000000000000000, 0.9876883405951377704, 1.000000000000000000, 0.9876883405951377704, 1.000000000000000000, 0.9876883405951377704, 1.000000000000000000, 0.9876883405951377704, 1.000000000000000000, 0.9876883405951377704, 1.000000000000000000, 0.9876883405951377704, 1.000000000000000000) ) ) 
 REPRESENTATION_ITEM ( '' )  SURFACE ( )  );
#6275=CARTESIAN_POINT ( 'NONE',  ( 10.00000000000000533, 1.185096637661293251, -5.575441324182679459 ) ) ;
#6276=CARTESIAN_POINT ( 'NONE',  ( 13.84374999795161543, 0.5109457054262118714, -4.861323657744403448 ) ) ;
#6277=EDGE_CURVE ( 'NONE', #2859, #5462, #17797, .T. ) ;
#6278=DIRECTION ( 'NONE',  ( -1.000000000000000000, 0.000000000000000000, 0.000000000000000000 ) ) ;
#6279=LINE ( 'NONE', #12404, #7132 ) ;
#6281=CARTESIAN_POINT ( 'NONE',  ( 14.46874999795161720, 2.873153789725825913, 3.954556930911861112 ) ) ;
#6283=VERTEX_POINT ( 'NONE', #15687 ) ;
#6286=FACE_OUTER_BOUND ( 'NONE', #4487, .T. ) ;
#6297=ORIENTED_EDGE ( 'NONE', *, *, #8769, .T. ) ;
#6298=CIRCLE ( 'NONE', #7573, 5.700000000000001954 ) ;
#6302=CARTESIAN_POINT ( 'NONE',  ( 11.50000000000000355, -3.631840208645826351, 4.484949146646356688 ) ) ;
#6303=ORIENTED_EDGE ( 'NONE', *, *, #18715, .F. ) ;
#6307=DIRECTION ( 'NONE',  ( -1.000000000000000000, -0.000000000000000000, -0.000000000000000000 ) ) ;
#6311=EDGE_CURVE ( 'NONE', #7195, #3069, #1166, .T. ) ;
#6319=CARTESIAN_POINT ( 'NONE',  ( 6.000000000000005329, 0.000000000000000000, 0.000000000000000000 ) ) ;
#6322=EDGE_CURVE ( 'NONE', #5554, #17466, #17286, .T. ) ;
#6328=FACE_OUTER_BOUND ( 'NONE', #9235, .T. ) ;
#6334=CARTESIAN_POINT ( 'NONE',  ( 13.46874999795161543, -0.5109457054261780096, 4.861323657744406113 ) ) ;
#6339=ORIENTED_EDGE ( 'NONE', *, *, #6539, .F. ) ;
#6340=EDGE_CURVE ( 'NONE', #2660, #5462, #3794, .T. ) ;
#6341=EDGE_CURVE ( 'NONE', #18865, #3717, #5452, .T. ) ;
#6349=VECTOR ( 'NONE', #5450, 1000.000000000000000 ) ;
#6353=ORIENTED_EDGE ( 'NONE', *, *, #10065, .F. ) ;
#6361=CARTESIAN_POINT ( 'NONE',  ( 6.000000000000005329, 0.000000000000000000, 0.000000000000000000 ) ) ;
#6362=CARTESIAN_POINT ( 'NONE',  ( 9.343749997951615427, -3.499494075959840966, 3.499494075959792116 ) ) ;
#6366=EDGE_CURVE ( 'NONE', #14247, #18527, #7554, .T. ) ;
#6371=FACE_OUTER_BOUND ( 'NONE', #534, .T. ) ;
#6374=CARTESIAN_POINT ( 'NONE',  ( 9.500000000000003553, 5.142044285764749922, -2.620002426024544473 ) ) ;
#6379=CARTESIAN_POINT ( 'NONE',  ( 12.00000000000000533, 1.185096637661215757, 5.575441324182695446 ) ) ;
#6389=CARTESIAN_POINT ( 'NONE',  ( 9.000000000000005329, -0.5958122406255588199, -5.668774803599165857 ) ) ;
#6398=EDGE_CURVE ( 'NONE', #6283, #8351, #17164, .T. ) ;
#6403=VERTEX_POINT ( 'NONE', #5464 ) ;
#6422=CARTESIAN_POINT ( 'NONE',  ( 2.999999999999998224, 0.000000000000000000, 0.000000000000000000 ) ) ;
#6461=CARTESIAN_POINT ( 'NONE',  ( 14.00000000000000533, 5.668774803599165857, -0.5958122406255597081 ) ) ;
#6463=AXIS2_PLACEMENT_3D ( 'NONE', #18064, #2541, #14960 ) ;
#6464=LINE ( 'NONE', #593, #3256 ) ;
#6468=EDGE_LOOP ( 'NONE', ( #17204, #1647, #11480, #15460 ) ) ;
#6479=CARTESIAN_POINT ( 'NONE',  ( 11.46874999795161543, 2.444050593749990785, 4.233219804643887585 ) ) ;
#6487=ORIENTED_EDGE ( 'NONE', *, *, #6277, .F. ) ;
#6488=CARTESIAN_POINT ( 'NONE',  ( 13.34374999795161365, -4.409619785863891472, -2.246813503491864150 ) ) ;
#6496=CARTESIAN_POINT ( 'NONE',  ( 8.312499995903225525, 1.761396867937200517, -5.421022142882375938 ) ) ;
#6504=( BOUNDED_CURVE ( )  B_SPLINE_CURVE ( 2, ( #7764, #13877, #1569, #6252, #12378, #555, #12751, #5132, #11246, #10245, #2717, #8834, #14838, #4131, #5618 ),
 .UNSPECIFIED., .F., .F. ) 
 B_SPLINE_CURVE_WITH_KNOTS ( ( 3, 2, 2, 2, 2, 2, 2, 3 ),
 ( 0.000000000000000000, 0.05000000000000000278, 0.1000000000000000056, 0.1499999999999999944, 0.2000000000000000111, 0.2500000000000000000, 0.2999999999999999889, 0.3078686208676164604 ),
 .UNSPECIFIED. ) 
 CURVE ( )  GEOMETRIC_REPRESENTATION_ITEM ( )  RATIONAL_B_SPLINE_CURVE ( ( 1.000000000000000000, 0.9876883405951377704, 1.000000000000000000, 0.9876883405951377704, 1.000000000000000000, 0.9876883405951377704, 1.000000000000000000, 0.9876883405951377704, 1.000000000000000000, 0.9876883405951377704, 1.000000000000000000, 0.9876883405951377704, 1.000000000000000000, 0.9980624843978382899, 0.9967347918236166837 ) ) 
 REPRESENTATION_ITEM ( '' )  );
#6523=CARTESIAN_POINT ( 'NONE',  ( 6.500000000000005329, -5.387740456496247887, 2.068159791354145849 ) ) ;
#6524=CARTESIAN_POINT ( 'NONE',  ( 13.31249999590322730, 4.235925505221192822, -3.814044456245444081 ) ) ;
#6536=CARTESIAN_POINT ( 'NONE',  ( 11.46874999795161543, -2.444050593750019651, 4.233219804643871598 ) ) ;
#6539=EDGE_CURVE ( 'NONE', #9343, #16572, #19052, .T. ) ;
#6543=ADVANCED_FACE ( 'NONE', ( #19438 ), #5341, .F. ) ;
#6569=CARTESIAN_POINT ( 'NONE',  ( 7.843749997951614539, 4.781284448697194378, -1.016293382781411569 ) ) ;
#6577=CARTESIAN_POINT ( 'NONE',  ( 6.500000000000005329, 5.387740456496233676, -2.068159791354183596 ) ) ;
#6586=CARTESIAN_POINT ( 'NONE',  ( 8.812499995903225525, -2.620002426024580000, 5.142044285764733935 ) ) ;
#6592=CARTESIAN_POINT ( 'NONE',  ( 12.99999999999969980, 5.254364458093119694, 1.428050399360184963 ) ) ;
#6594=ORIENTED_EDGE ( 'NONE', *, *, #4568, .F. ) ;
#6622=CARTESIAN_POINT ( 'NONE',  ( 9.812499995903223748, -1.493657965219446382, -5.574407415329178939 ) ) ;
#6627=ORIENTED_EDGE ( 'NONE', *, *, #3744, .T. ) ;
#6630=CARTESIAN_POINT ( 'NONE',  ( 9.843749997951615427, 4.465502636338023912, 1.988169868018593300 ) ) ;
#6635=CARTESIAN_POINT ( 'NONE',  ( 12.46874999795161543, -3.632567103900546712, 3.270778111535314281 ) ) ;
#6660=CARTESIAN_POINT ( 'NONE',  ( 11.34374999795161543, 1.773574444220790136, -4.620319390059805187 ) ) ;
#6661=CARTESIAN_POINT ( 'NONE',  ( 9.843749997951615427, -3.954556930911881985, 2.873153789725797491 ) ) ;
#6664=CARTESIAN_POINT ( 'NONE',  ( 7.000000000000005329, 1.761396867937200517, -5.421022142882375938 ) ) ;
#6677=CARTESIAN_POINT ( 'NONE',  ( 12.65441706489329299, 2.315350974882481871, 5.245024560144870840 ) ) ;
#6680=CARTESIAN_POINT ( 'NONE',  ( 12.46874999795161543, -3.632567103900546712, 3.270778111535314281 ) ) ;
#6681=CARTESIAN_POINT ( 'NONE',  ( 9.843749997951615427, -4.465502636338009701, -1.988169868018624609 ) ) ;
#6687=CARTESIAN_POINT ( 'NONE',  ( 10.81249999590322375, -5.142044285764769462, 2.620002426024508502 ) ) ;
#6689=AXIS2_PLACEMENT_3D ( 'NONE', #11337, #17435, #3723 ) ;
#6694=CARTESIAN_POINT ( 'NONE',  ( 11.81249999590322552, 5.700000000000000178, -0.9027913098498572264 ) ) ;
#6701=CARTESIAN_POINT ( 'NONE',  ( 10.46874999795161720, -4.648860486681964055, 1.510506337161829027 ) ) ;
#6706=PLANE ( 'NONE',  #6689 ) ;
#6708=DIRECTION ( 'NONE',  ( 0.000000000000000000, -0.7315216790650492795, 0.6818181818181815457 ) ) ;
#6727=CARTESIAN_POINT ( 'NONE',  ( 11.84374999795161365, -2.444050593750019651, 4.233219804643871598 ) ) ;
#6764=CARTESIAN_POINT ( 'NONE',  ( 13.00000000000000178, -3.830176896397409880, 3.037670790816764388 ) ) ;
#6774=DIRECTION ( 'NONE',  ( -1.000000000000000000, -0.000000000000000000, -0.000000000000000000 ) ) ;
#6788=CARTESIAN_POINT ( 'NONE',  ( 6.234374998975811266, 0.000000000000000000, -5.294050593750000644 ) ) ;
#6793=AXIS2_PLACEMENT_3D ( 'NONE', #10555, #4739, #10656 ) ;
#6797=ORIENTED_EDGE ( 'NONE', *, *, #7445, .T. ) ;
#6804=ORIENTED_EDGE ( 'NONE', *, *, #18367, .T. ) ;
#6834=ORIENTED_EDGE ( 'NONE', *, *, #6398, .F. ) ;
#6836=DIRECTION ( 'NONE',  ( -1.000000000000000000, -0.000000000000000000, -0.000000000000000000 ) ) ;
#6837=CARTESIAN_POINT ( 'NONE',  ( 10.81249999590322375, -5.142044285764769462, 2.620002426024508502 ) ) ;
#6838=CARTESIAN_POINT ( 'NONE',  ( 7.968749997951616315, 2.695436003842704764, 4.150607464521811174 ) ) ;
#6846=CARTESIAN_POINT ( 'NONE',  ( 12.00000000000000533, -5.421022142882365280, -1.761396867937238042 ) ) ;
#6850=ORIENTED_EDGE ( 'NONE', *, *, #7039, .F. ) ;
#6858=CARTESIAN_POINT ( 'NONE',  ( 6.968749997951614539, -3.846120219227901149, -3.114526743279308896 ) ) ;
#6859=CARTESIAN_POINT ( 'NONE',  ( 13.00000000000000888, -4.496324317583046515, -1.917446440021278731 ) ) ;
#6865=DIRECTION ( 'NONE',  ( -1.000000000000000000, -0.000000000000000000, -0.000000000000000000 ) ) ;
#6878=CARTESIAN_POINT ( 'NONE',  ( 12.84374999795161543, -1.016293382781378485, -4.781284448697201483 ) ) ;
#6882=CARTESIAN_POINT ( 'NONE',  ( 8.343749997951611874, -2.246813503491864150, 4.409619785863891472 ) ) ;
#6883=DIRECTION ( 'NONE',  ( 0.000000000000000000, 3.552713678800500929E-15, 1.000000000000000000 ) ) ;
#6896=VERTEX_POINT ( 'NONE', #8527 ) ;
#6899=CARTESIAN_POINT ( 'NONE',  ( 8.312499995903225525, -5.575441324182703440, 1.185096637661176677 ) ) ;
#6900=CIRCLE ( 'NONE', #9480, 4.400000000000000355 ) ;
#6910=CARTESIAN_POINT ( 'NONE',  ( 12.31249999590322552, -2.850000000000023626, 4.936344801571289409 ) ) ;
#6922=ADVANCED_FACE ( 'NONE', ( #19126 ), #8326, .T. ) ;
#6931=EDGE_LOOP ( 'NONE', ( #6487, #8119, #2632, #4055 ) ) ;
#6965=CARTESIAN_POINT ( 'NONE',  ( 10.84374999795161543, 3.632567103900524064, 3.270778111535338262 ) ) ;
#6996=CARTESIAN_POINT ( 'NONE',  ( 9.812499995903225525, -5.574407415329147852, -1.493657965219562511 ) ) ;
#7002=CIRCLE ( 'NONE', #12141, 5.700000000000001954 ) ;
#7007=VERTEX_POINT ( 'NONE', #16228 ) ;
#7033=CARTESIAN_POINT ( 'NONE',  ( 13.00000000000000000, 0.2080849974989116558, 4.883670121236158401 ) ) ;
#7035=VERTEX_POINT ( 'NONE', #10423 ) ;
#7039=EDGE_CURVE ( 'NONE', #2859, #17179, #13227, .T. ) ;
#7064=AXIS2_PLACEMENT_3D ( 'NONE', #16835, #16732, #6108 ) ;
#7086=CARTESIAN_POINT ( 'NONE',  ( 7.500000000000005329, -2.620002426024580000, 5.142044285764733935 ) ) ;
#7098=CARTESIAN_POINT ( 'NONE',  ( 6.843749997951615427, -3.413342815706642518E-14, 4.888101187500000222 ) ) ;
#7104=EDGE_CURVE ( 'NONE', #19695, #2660, #15253, .T. ) ;
#7109=CARTESIAN_POINT ( 'NONE',  ( 13.00000000000000533, 5.207209108562852684, -2.318398865532001363 ) ) ;
#7111=CARTESIAN_POINT ( 'NONE',  ( 7.968749997951616315, 2.246813503491833508, -4.409619785863906571 ) ) ;
#7132=VECTOR ( 'NONE', #7881, 1000.000000000000000 ) ;
#7149=CARTESIAN_POINT ( 'NONE',  ( 13.00000000000000178, -4.390212428369197006, -2.150226904532469341 ) ) ;
#7155=CARTESIAN_POINT ( 'NONE',  ( 14.34374999795161365, 3.499494075959816541, 3.499494075959815653 ) ) ;
#7156=CARTESIAN_POINT ( 'NONE',  ( 9.843749997951615427, 4.465502636338024800, 1.988169868018593300 ) ) ;
#7163=AXIS2_PLACEMENT_3D ( 'NONE', #3031, #15450, #4442 ) ;
#7175=CARTESIAN_POINT ( 'NONE',  ( 11.31249999590322375, -4.235925505221111997, -3.814044456245531567 ) ) ;
#7181=CARTESIAN_POINT ( 'NONE',  ( 7.468749997951615427, 1.510506337161861445, -4.648860486681953397 ) ) ;
#7184=CARTESIAN_POINT ( 'NONE',  ( 6.500000000000005329, -0.9027913098498965283, 5.699999999999994849 ) ) ;
#7188=CARTESIAN_POINT ( 'NONE',  ( 10.46874999795161720, -4.648860486681964055, 1.510506337161829027 ) ) ;
#7195=VERTEX_POINT ( 'NONE', #18608 ) ;
#7207=VECTOR ( 'NONE', #15790, 1000.000000000000000 ) ;
#7216=CARTESIAN_POINT ( 'NONE',  ( 7.000000000000005329, -5.575441324182703440, 1.185096637661176677 ) ) ;
#7239=CARTESIAN_POINT ( 'NONE',  ( 14.00000000000000533, -5.668774803599162304, 0.5958122406255995651 ) ) ;
#7252=CARTESIAN_POINT ( 'NONE',  ( 6.843749997951615427, 0.000000000000000000, -4.888101187500000222 ) ) ;
#7255=FILL_AREA_STYLE ('',( #17993 ) ) ;
#7265=CARTESIAN_POINT ( 'NONE',  ( 0.000000000000000000, 0.000000000000000000, 5.700000000000001954 ) ) ;
#7272=CARTESIAN_POINT ( 'NONE',  ( 10.96874999795161720, 1.773574444220790136, -4.620319390059805187 ) ) ;
#7288=CARTESIAN_POINT ( 'NONE',  ( 13.84374999795161543, 3.954556930911862000, 2.873153789725825025 ) ) ;
#7294=FACE_OUTER_BOUND ( 'NONE', #682, .T. ) ;
#7301=ORIENTED_EDGE ( 'NONE', *, *, #6398, .T. ) ;
#7303=CARTESIAN_POINT ( 'NONE',  ( 11.84374999795161365, 2.444050593749991229, 4.233219804643887585 ) ) ;
#7308=DIRECTION ( 'NONE',  ( 0.000000000000000000, 0.000000000000000000, 1.000000000000000000 ) ) ;
#7314=( BOUNDED_CURVE ( )  B_SPLINE_CURVE ( 2, ( #12791, #8387, #6664, #18059, #12890, #13261, #2079, #18989, #11953, #2279, #14291, #18888, #5281, #11390, #8283 ),
 .UNSPECIFIED., .F., .F. ) 
 B_SPLINE_CURVE_WITH_KNOTS ( ( 3, 2, 2, 2, 2, 2, 2, 3 ),
 ( 0.000000000000000000, 0.04999999999999999584, 0.09999999999999999167, 0.1499999999999999944, 0.1999999999999999833, 0.2500000000000000000, 0.2999999999999999889, 0.3499999999999999778 ),
 .UNSPECIFIED. ) 
 CURVE ( )  GEOMETRIC_REPRESENTATION_ITEM ( )  RATIONAL_B_SPLINE_CURVE ( ( 1.000000000000000000, 0.9876883405951377704, 1.000000000000000000, 0.9876883405951377704, 1.000000000000000000, 0.9876883405951377704, 1.000000000000000000, 0.9876883405951377704, 1.000000000000000000, 0.9876883405951377704, 1.000000000000000000, 0.9876883405951377704, 1.000000000000000000, 0.9876883405951377704, 1.000000000000000000 ) ) 
 REPRESENTATION_ITEM ( '' )  );
#7316=CARTESIAN_POINT ( 'NONE',  ( 10.00000000000000533, -4.235925505221111997, -3.814044456245531567 ) ) ;
#7328=CARTESIAN_POINT ( 'NONE',  ( 13.00000000000000533, -4.611396867937178179, -3.350375938067128967 ) ) ;
#7340=CARTESIAN_POINT ( 'NONE',  ( 9.500000000000003553, -0.3020334839682879413, 5.763142191869155440 ) ) ;
#7372=CARTESIAN_POINT ( 'NONE',  ( 13.84374999795161543, -4.465502636338038123, 1.988169868018562880 ) ) ;
#7373=CARTESIAN_POINT ( 'NONE',  ( 10.31249999590322552, -5.207209108562803834, -2.318398865532109721 ) ) ;
#7379=CARTESIAN_POINT ( 'NONE',  ( 11.96874999795161365, 4.888101187500000222, 0.7741991708318884946 ) ) ;
#7387=CARTESIAN_POINT ( 'NONE',  ( 14.46874999795161720, 2.873153789725825913, 3.954556930911861112 ) ) ;
#7389=DIRECTION ( 'NONE',  ( 0.000000000000000000, 1.000000000000000000, 6.982962677686267499E-15 ) ) ;
#7403=CARTESIAN_POINT ( 'NONE',  ( 11.31249999590322375, 4.235925505221138643, 3.814044456245502701 ) ) ;
#7415=CARTESIAN_POINT ( 'NONE',  ( 11.50000000000000355, -2.068159791354146293, -5.387740456496247887 ) ) ;
#7443=ORIENTED_EDGE ( 'NONE', *, *, #4043, .T. ) ;
#7445=EDGE_CURVE ( 'NONE', #2779, #1853, #10202, .T. ) ;
#7461=( NAMED_UNIT ( * ) SI_UNIT ( $, .STERADIAN. ) SOLID_ANGLE_UNIT ( ) );
#7473=ADVANCED_FACE ( 'NONE', ( #13388 ), #5877, .T. ) ;
#7480=EDGE_CURVE ( 'NONE', #16413, #17840, #19388, .T. ) ;
#7483=CARTESIAN_POINT ( 'NONE',  ( 9.500000000000005329, 4.840010801796481132, 3.143139765844623401 ) ) ;
#7492=CARTESIAN_POINT ( 'NONE',  ( 9.468749997951615427, 0.5109457054261445919, 4.861323657744411442 ) ) ;
#7493=CARTESIAN_POINT ( 'NONE',  ( 11.46874999795161543, -4.888101187500000222, -3.383411828340740850E-14 ) ) ;
#7494=CARTESIAN_POINT ( 'NONE',  ( 7.468749997951615427, 1.510506337161861445, -4.648860486681953397 ) ) ;
#7506=EDGE_LOOP ( 'NONE', ( #18358, #4666 ) ) ;
#7508=CARTESIAN_POINT ( 'NONE',  ( 14.81249999590322552, -1.493657965219523209, 5.574407415329156734 ) ) ;
#7520=CARTESIAN_POINT ( 'NONE',  ( 14.00000000000000533, 2.318398865532109276, -5.207209108562804722 ) ) ;
#7554=( BOUNDED_CURVE ( )  B_SPLINE_CURVE ( 2, ( #2461, #4074, #14687, #3776, #19272, #15890, #2275, #14591, #10182, #14390, #13081, #8574, #12887, #18983, #19079 ),
 .UNSPECIFIED., .F., .F. ) 
 B_SPLINE_CURVE_WITH_KNOTS ( ( 3, 2, 2, 2, 2, 2, 2, 3 ),
 ( 0.000000000000000000, 0.05000000000000000278, 0.1000000000000000056, 0.1499999999999999944, 0.2000000000000000111, 0.2500000000000000000, 0.2999999999999999889, 0.3078686208676164604 ),
 .UNSPECIFIED. ) 
 CURVE ( )  GEOMETRIC_REPRESENTATION_ITEM ( )  RATIONAL_B_SPLINE_CURVE ( ( 1.000000000000000000, 0.9876883405951377704, 1.000000000000000000, 0.9876883405951377704, 1.000000000000000000, 0.9876883405951377704, 1.000000000000000000, 0.9876883405951377704, 1.000000000000000000, 0.9876883405951377704, 1.000000000000000000, 0.9876883405951377704, 1.000000000000000000, 0.9980624843978382899, 0.9967347918236166837 ) ) 
 REPRESENTATION_ITEM ( '' )  );
#7559=CARTESIAN_POINT ( 'NONE',  ( 7.843749997951614539, 1.510506337161861445, -4.648860486681953397 ) ) ;
#7573=AXIS2_PLACEMENT_3D ( 'NONE', #9841, #2314, #17624 ) ;
#7574=CARTESIAN_POINT ( 'NONE',  ( 12.99999999999999467, 4.390212428369212105, 2.150226904532439143 ) ) ;
#7580=CARTESIAN_POINT ( 'NONE',  ( 12.81249999590322552, -3.631840208645826351, 4.484949146646356688 ) ) ;
#7581=CARTESIAN_POINT ( 'NONE',  ( 13.81249999590322552, -0.3020334839682081163, -5.763142191869158992 ) ) ;
#7582=DIRECTION ( 'NONE',  ( 1.000000000000000000, 0.000000000000000000, 0.000000000000000000 ) ) ;
#7587=CARTESIAN_POINT ( 'NONE',  ( 12.96874999795161543, 4.409619785863906571, 2.246813503491833508 ) ) ;
#7595=DIRECTION ( 'NONE',  ( -1.000000000000000000, 0.000000000000000000, 0.000000000000000000 ) ) ;
#7597=CARTESIAN_POINT ( 'NONE',  ( 8.343749997951611874, 2.246813503491833508, -4.409619785863906571 ) ) ;
#7612=CARTESIAN_POINT ( 'NONE',  ( 12.81249999590322552, 2.068159791354184485, 5.387740456496232788 ) ) ;
#7625=CARTESIAN_POINT ( 'NONE',  ( 13.00000000000000000, 0.2705398332808751638, 4.881009025374877908 ) ) ;
#7631=CARTESIAN_POINT ( 'NONE',  ( -2.000000000000001776, -3.950217066951267952, 3.681818181818181213 ) ) ;
#7648=ORIENTED_EDGE ( 'NONE', *, *, #9847, .T. ) ;
#7656=DIRECTION ( 'NONE',  ( 0.000000000000000000, -0.5000000000000098810, 0.8660254037844330455 ) ) ;
#7658=LINE ( 'NONE', #1275, #18348 ) ;
#7664=( LENGTH_UNIT ( ) NAMED_UNIT ( * ) SI_UNIT ( .MILLI., .METRE. ) );
#7666=ORIENTED_EDGE ( 'NONE', *, *, #2536, .F. ) ;
#7679=ORIENTED_EDGE ( 'NONE', *, *, #18251, .T. ) ;
#7680=CARTESIAN_POINT ( 'NONE',  ( 12.46874999795161543, 3.632567103900569361, -3.270778111535288080 ) ) ;
#7682=CARTESIAN_POINT ( 'NONE',  ( 14.34374999795161365, 1.280903732194486722, -4.780397808154247308 ) ) ;
#7687=CARTESIAN_POINT ( 'NONE',  ( 8.000000000000005329, 3.350375938067097437, -4.611396867937201272 ) ) ;
#7701=CARTESIAN_POINT ( 'NONE',  ( 11.96874999795161365, -4.888101187499994893, -0.7741991708319226895 ) ) ;
#7707=AXIS2_PLACEMENT_3D ( 'NONE', #2607, #18035, #18228 ) ;
#7714=CARTESIAN_POINT ( 'NONE',  ( 10.46874999795161720, 4.648860486681953397, -1.510506337161861667 ) ) ;
#7737=VECTOR ( 'NONE', #10214, 1000.000000000000000 ) ;
#7750=EDGE_CURVE ( 'NONE', #18923, #18527, #14834, .T. ) ;
#7752=ORIENTED_EDGE ( 'NONE', *, *, #14032, .F. ) ;
#7755=CARTESIAN_POINT ( 'NONE',  ( 6.468749997951615427, 4.233219804643871598, 2.444050593750020095 ) ) ;
#7764=CARTESIAN_POINT ( 'NONE',  ( 6.843749997951615427, 4.233219804643871598, 2.444050593750020095 ) ) ;
#7781=DIRECTION ( 'NONE',  ( -1.000000000000000000, 0.000000000000000000, 0.000000000000000000 ) ) ;
#7782=CARTESIAN_POINT ( 'NONE',  ( 13.00000000000000000, -4.333424887442987483, -2.261628166637620119 ) ) ;
#7785=CARTESIAN_POINT ( 'NONE',  ( 8.343749997951611874, -4.942249507334558700, 0.2590123213420631454 ) ) ;
#7791=CARTESIAN_POINT ( 'NONE',  ( 12.46874999795161543, 4.648860486681953397, 1.510506337161861223 ) ) ;
#7798=CARTESIAN_POINT ( 'NONE',  ( 13.50000000000000533, -1.493657965219523209, 5.574407415329156734 ) ) ;
#7808=ADVANCED_BREP_SHAPE_REPRESENTATION ( '', ( #2634, #16724 ), #12592 ) ;
#7834=VERTEX_POINT ( 'NONE', #582 ) ;
#7836=CARTESIAN_POINT ( 'NONE',  ( 2.999999999999998224, 3.950217066951266176, 3.681818181818181213 ) ) ;
#7840=CARTESIAN_POINT ( 'NONE',  ( 13.00000000000000000, -0.2080849974988778772, -4.883670121236158401 ) ) ;
#7841=EDGE_LOOP ( 'NONE', ( #13790, #9790, #2797, #15626 ) ) ;
#7855=EDGE_CURVE ( 'NONE', #5327, #18865, #18206, .T. ) ;
#7881=DIRECTION ( 'NONE',  ( -1.000000000000000000, -0.000000000000000000, -0.000000000000000000 ) ) ;
#7892=FACE_OUTER_BOUND ( 'NONE', #12635, .T. ) ;
#7893=CARTESIAN_POINT ( 'NONE',  ( 10.00000000000000533, 4.235925505221138643, 3.814044456245502701 ) ) ;
#7900=CARTESIAN_POINT ( 'NONE',  ( 12.34374999795161543, -4.888101187499994893, -0.7741991708319226895 ) ) ;
#7915=( BOUNDED_SURFACE ( )  B_SPLINE_SURFACE ( 1, 2, ( 
 ( #13472, #19475, #13577, #4376, #19675, #1473, #4571, #19575, #1177, #12177, #16585, #14885, #11979, #9082, #15180, #17883, #8782 ),
 ( #7252, #17989, #7559, #16384, #10390, #2865, #13678, #16489, #18283, #5668, #10681, #16788, #1080, #15083, #2764, #7155, #19378 ) ),
 .UNSPECIFIED., .F., .F., .F. ) 
 B_SPLINE_SURFACE_WITH_KNOTS ( ( 2, 2 ),
 ( 3, 2, 2, 2, 2, 2, 2, 2, 3 ),
 ( 0.000000000000000000, 1.000000000000000000 ),
 ( 0.000000000000000000, 0.05000000000000000278, 0.1000000000000000056, 0.1499999999999999944, 0.2000000000000000111, 0.2500000000000000000, 0.2999999999999999889, 0.3499999999999999778, 0.4000000000000000222 ),
 .UNSPECIFIED. ) 
 GEOMETRIC_REPRESENTATION_ITEM ( )  RATIONAL_B_SPLINE_SURFACE ( (
 ( 1.000000000000000000, 0.9876883405951377704, 1.000000000000000000, 0.9876883405951377704, 1.000000000000000000, 0.9876883405951377704, 1.000000000000000000, 0.9876883405951377704, 1.000000000000000000, 0.9876883405951377704, 1.000000000000000000, 0.9876883405951377704, 1.000000000000000000, 0.9876883405951377704, 1.000000000000000000, 0.9876883405951377704, 1.000000000000000000),
 ( 1.000000000000000000, 0.9876883405951377704, 1.000000000000000000, 0.9876883405951377704, 1.000000000000000000, 0.9876883405951377704, 1.000000000000000000, 0.9876883405951377704, 1.000000000000000000, 0.9876883405951377704, 1.000000000000000000, 0.9876883405951377704, 1.000000000000000000, 0.9876883405951377704, 1.000000000000000000, 0.9876883405951377704, 1.000000000000000000) ) ) 
 REPRESENTATION_ITEM ( '' )  SURFACE ( )  );
#7925=LINE ( 'NONE', #14136, #19567 ) ;
#7935=CARTESIAN_POINT ( 'NONE',  ( 13.84374999795161543, 4.465502636338051445, -1.988169868018530906 ) ) ;
#7937=EDGE_LOOP ( 'NONE', ( #12356, #6834, #5145, #5339, #12057 ) ) ;
#7943=CARTESIAN_POINT ( 'NONE',  ( 12.46874999795161543, 1.016293382781411792, 4.781284448697194378 ) ) ;
#7978=CARTESIAN_POINT ( 'NONE',  ( 11.84374999795161365, -2.444050593749961031, -4.233219804643904460 ) ) ;
#7983=CARTESIAN_POINT ( 'NONE',  ( 7.343749997951615427, 4.620319390059830056, -1.773574444220725521 ) ) ;
#8001=CARTESIAN_POINT ( 'NONE',  ( 13.00000000000000000, 3.840809689103004576, -4.211671987713725862 ) ) ;
#8020=DIRECTION ( 'NONE',  ( -1.000000000000000000, 0.000000000000000000, 0.000000000000000000 ) ) ;
#8029=ORIENTED_EDGE ( 'NONE', *, *, #11239, .F. ) ;
#8031=ADVANCED_FACE ( 'NONE', ( #2929 ), #9045, .F. ) ;
#8038=CARTESIAN_POINT ( 'NONE',  ( -0.000000000000000000, 0.000000000000000000, 0.000000000000000000 ) ) ;
#8064=ORIENTED_EDGE ( 'NONE', *, *, #10080, .T. ) ;
#8077=CARTESIAN_POINT ( 'NONE',  ( 11.84374999795161365, -4.888101187500000222, -3.383411828340740850E-14 ) ) ;
#8093=DIRECTION ( 'NONE',  ( -1.000000000000000000, 0.000000000000000000, 0.000000000000000000 ) ) ;
#8103=EDGE_CURVE ( 'NONE', #5554, #16744, #18304, .T. ) ;
#8104=CARTESIAN_POINT ( 'NONE',  ( 13.00000000000000533, 5.207209108562852684, -2.318398865532001363 ) ) ;
#8107=ORIENTED_EDGE ( 'NONE', *, *, #12498, .F. ) ;
#8111=CARTESIAN_POINT ( 'NONE',  ( 10.00000000000000533, -1.185096637661254171, 5.575441324182689229 ) ) ;
#8119=ORIENTED_EDGE ( 'NONE', *, *, #12718, .F. ) ;
#8120=EDGE_CURVE ( 'NONE', #19560, #15, #7925, .T. ) ;
#8136=EDGE_CURVE ( 'NONE', #17840, #13931, #12558, .T. ) ;
#8140=CARTESIAN_POINT ( 'NONE',  ( 12.50000000000000533, -0.3020334839682081163, -5.763142191869158992 ) ) ;
#8141=CARTESIAN_POINT ( 'NONE',  ( 7.312499995903225525, -4.936344801571268093, -2.850000000000058265 ) ) ;
#8144=CARTESIAN_POINT ( 'NONE',  ( 13.00000000000000533, 0.2990843904630375860, -5.438532396800193958 ) ) ;
#8151=DIRECTION ( 'NONE',  ( -1.000000000000000000, 0.000000000000000000, 0.000000000000000000 ) ) ;
#8155=CARTESIAN_POINT ( 'NONE',  ( 8.468749997951615427, 1.988169868018562436, 4.465502636338039011 ) ) ;
#8156=VERTEX_POINT ( 'NONE', #3729 ) ;
#8178=CARTESIAN_POINT ( 'NONE',  ( 12.84374999795161543, 3.632567103900569361, -3.270778111535288080 ) ) ;
#8191=EDGE_CURVE ( 'NONE', #17466, #11664, #16708, .T. ) ;
#8206=CARTESIAN_POINT ( 'NONE',  ( 7.343749997951615427, -0.7741991708319229115, 4.888101187499994893 ) ) ;
#8210=CARTESIAN_POINT ( 'NONE',  ( 7.078124996927420476, 4.584782303107598267, -2.647025296874989664 ) ) ;
#8211=CARTESIAN_POINT ( 'NONE',  ( 12.00000000000000533, -4.235925505221167064, 3.814044456245474279 ) ) ;
#8212=( BOUNDED_SURFACE ( )  B_SPLINE_SURFACE ( 1, 2, ( 
 ( #15102, #16506, #10599, #15202, #4197, #16604, #4295, #11899, #8698, #16704, #4488, #7580, #13394, #10310, #13597, #15002, #19295 ),
 ( #11800, #1293, #18012, #2988, #2784, #13297, #5780, #9102, #19397, #1399, #5979, #1494, #2884, #8999, #7372, #5587, #8899 ) ),
 .UNSPECIFIED., .F., .F., .F. ) 
 B_SPLINE_SURFACE_WITH_KNOTS ( ( 2, 2 ),
 ( 3, 2, 2, 2, 2, 2, 2, 2, 3 ),
 ( 0.000000000000000000, 1.000000000000000000 ),
 ( 0.000000000000000000, 0.05000000000000000278, 0.1000000000000000056, 0.1499999999999999944, 0.2000000000000000111, 0.2500000000000000000, 0.2999999999999999889, 0.3499999999999999778, 0.4000000000000000222 ),
 .UNSPECIFIED. ) 
 GEOMETRIC_REPRESENTATION_ITEM ( )  RATIONAL_B_SPLINE_SURFACE ( (
 ( 1.000000000000000000, 0.9876883405951377704, 1.000000000000000000, 0.9876883405951377704, 1.000000000000000000, 0.9876883405951377704, 1.000000000000000000, 0.9876883405951377704, 1.000000000000000000, 0.9876883405951377704, 1.000000000000000000, 0.9876883405951377704, 1.000000000000000000, 0.9876883405951377704, 1.000000000000000000, 0.9876883405951377704, 1.000000000000000000),
 ( 1.000000000000000000, 0.9876883405951377704, 1.000000000000000000, 0.9876883405951377704, 1.000000000000000000, 0.9876883405951377704, 1.000000000000000000, 0.9876883405951377704, 1.000000000000000000, 0.9876883405951377704, 1.000000000000000000, 0.9876883405951377704, 1.000000000000000000, 0.9876883405951377704, 1.000000000000000000, 0.9876883405951377704, 1.000000000000000000) ) ) 
 REPRESENTATION_ITEM ( '' )  SURFACE ( )  );
#8232=ADVANCED_FACE ( 'NONE', ( #19513 ), #16622, .T. ) ;
#8243=CARTESIAN_POINT ( 'NONE',  ( 13.00000000000000178, -0.3329550909586923013, -4.877148943244129953 ) ) ;
#8244=ORIENTED_EDGE ( 'NONE', *, *, #9382, .T. ) ;
#8251=CARTESIAN_POINT ( 'NONE',  ( 7.343749997951615427, 4.620319390059829168, -1.773574444220725077 ) ) ;
#8255=CARTESIAN_POINT ( 'NONE',  ( 6.500000000000005329, 4.484949146646356688, 3.631840208645826795 ) ) ;
#8283=CARTESIAN_POINT ( 'NONE',  ( 13.00000000000000533, 4.611396867937201272, 3.350375938067096548 ) ) ;
#8295=DIRECTION ( 'NONE',  ( 0.000000000000000000, 0.000000000000000000, 1.000000000000000000 ) ) ;
#8297=CARTESIAN_POINT ( 'NONE',  ( 11.84374999795161365, -2.444050593749961031, -4.233219804643904460 ) ) ;
#8302=ORIENTED_EDGE ( 'NONE', *, *, #8120, .F. ) ;
#8303=CARTESIAN_POINT ( 'NONE',  ( 14.34374999795161365, -3.499494075959791672, -3.499494075959840078 ) ) ;
#8319=CARTESIAN_POINT ( 'NONE',  ( 13.00000000000000000, 1.727010089215937905, 5.432074755721460591 ) ) ;
#8325=ADVANCED_FACE ( 'NONE', ( #7294 ), #10387, .F. ) ;
#8326=PLANE ( 'NONE',  #11890 ) ;
#8344=EDGE_CURVE ( 'NONE', #18748, #7195, #63, .T. ) ;
#8348=CARTESIAN_POINT ( 'NONE',  ( 7.343749997951615427, 3.846120219227923798, 3.114526743279282694 ) ) ;
#8351=VERTEX_POINT ( 'NONE', #8001 ) ;
#8361=ORIENTED_EDGE ( 'NONE', *, *, #703, .F. ) ;
#8362=B_SPLINE_CURVE_WITH_KNOTS ( 'NONE', 3,
 ( #15806, #10910, #18802, #14010 ),
 .UNSPECIFIED., .F., .F.,
 ( 4, 4 ),
 ( 0.000000000000000000, 0.001126652051248517921 ),
 .UNSPECIFIED. ) ;
#8365=EDGE_CURVE ( 'NONE', #2569, #16939, #12426, .T. ) ;
#8376=CARTESIAN_POINT ( 'NONE',  ( 13.00000000000000178, 3.947414994554159229, -2.883678330714892990 ) ) ;
#8380=ORIENTED_EDGE ( 'NONE', *, *, #4395, .T. ) ;
#8381=CARTESIAN_POINT ( 'NONE',  ( 10.46874999795161720, 1.016293382781477961, -4.781284448697179279 ) ) ;
#8383=CARTESIAN_POINT ( 'NONE',  ( 13.00000000000000178, -4.416988234087956045, -2.093740232017208935 ) ) ;
#8387=CARTESIAN_POINT ( 'NONE',  ( 6.500000000000005329, 0.9027913098498568933, -5.700000000000000178 ) ) ;
#8390=DIRECTION ( 'NONE',  ( 0.000000000000000000, 0.000000000000000000, 1.000000000000000000 ) ) ;
#8398=CARTESIAN_POINT ( 'NONE',  ( 13.00000000000000000, 1.727010089215937905, 5.432074755721460591 ) ) ;
#8403=ADVANCED_FACE ( 'NONE', ( #19010 ), #16399, .F. ) ;
#8405=CARTESIAN_POINT ( 'NONE',  ( 6.968749997951614539, -4.620319390059841602, 1.773574444220693103 ) ) ;
#8409=CARTESIAN_POINT ( 'NONE',  ( 12.34374999795161543, -4.888101187499994893, -0.7741991708319226895 ) ) ;
#8418=DIRECTION ( 'NONE',  ( -0.000000000000000000, 1.000000000000000000, 1.224646799147353207E-16 ) ) ;
#8420=ORIENTED_EDGE ( 'NONE', *, *, #19645, .T. ) ;
#8426=ORIENTED_EDGE ( 'NONE', *, *, #16149, .F. ) ;
#8427=CARTESIAN_POINT ( 'NONE',  ( 7.312499995903225525, -4.936344801571327601, 2.849999999999954348 ) ) ;
#8448=CARTESIAN_POINT ( 'NONE',  ( 6.843749997951615427, -4.233219804643852946, -2.444050593750049849 ) ) ;
#8454=ORIENTED_EDGE ( 'NONE', *, *, #8797, .F. ) ;
#8465=( BOUNDED_CURVE ( )  B_SPLINE_CURVE ( 2, ( #18210, #1593, #9107, #15209, #13602, #4397, #4299, #7483, #5889, #1404, #15107, #12770, #1298, #1498, #19700 ),
 .UNSPECIFIED., .F., .F. ) 
 B_SPLINE_CURVE_WITH_KNOTS ( ( 3, 2, 2, 2, 2, 2, 2, 3 ),
 ( 0.000000000000000000, 0.05000000000000000278, 0.1000000000000000056, 0.1499999999999999944, 0.2000000000000000111, 0.2500000000000000000, 0.2999999999999999889, 0.3333180920165871863 ),
 .UNSPECIFIED. ) 
 CURVE ( )  GEOMETRIC_REPRESENTATION_ITEM ( )  RATIONAL_B_SPLINE_CURVE ( ( 1.000000000000000000, 0.9876883405951377704, 1.000000000000000000, 0.9876883405951377704, 1.000000000000000000, 0.9876883405951377704, 1.000000000000000000, 0.9876883405951377704, 1.000000000000000000, 0.9876883405951377704, 1.000000000000000000, 0.9876883405951377704, 1.000000000000000000, 0.9917959799814384247, 0.9945256517182510247 ) ) 
 REPRESENTATION_ITEM ( '' )  );
#8485=CARTESIAN_POINT ( 'NONE',  ( 13.96874999795161365, 4.780397808154273065, -1.280903732194386802 ) ) ;
#8487=CARTESIAN_POINT ( 'NONE',  ( 11.81249999590322552, 2.068159791354258648, -5.387740456496205255 ) ) ;
#8495=CARTESIAN_POINT ( 'NONE',  ( 10.64522241986047568, 2.725425358843983450E-16, 5.700000000000002842 ) ) ;
#8500=CARTESIAN_POINT ( 'NONE',  ( 8.812499995903225525, 5.763142191869157216, -0.3020334839682480288 ) ) ;
#8503=CARTESIAN_POINT ( 'NONE',  ( 9.968749997951617203, -4.150607464521772094, -2.695436003842760275 ) ) ;
#8507=CARTESIAN_POINT ( 'NONE',  ( 12.50000000000000533, 4.840010801796527318, -3.143139765844555900 ) ) ;
#8527=CARTESIAN_POINT ( 'NONE',  ( 13.00000000000000000, 0.2080849974989116558, 4.883670121236158401 ) ) ;
#8546=CARTESIAN_POINT ( 'NONE',  ( 13.00000000000000178, -4.568735188514048140, -1.737869959597788672 ) ) ;
#8551=CARTESIAN_POINT ( 'NONE',  ( 10.31249999590322552, -4.611396867937225252, 3.350375938067065462 ) ) ;
#8561=DIRECTION ( 'NONE',  ( -1.000000000000000000, 0.000000000000000000, 0.000000000000000000 ) ) ;
#8563=CARTESIAN_POINT ( 'NONE',  ( 6.468749997951615427, -4.233219804643904460, 2.444050593749960587 ) ) ;
#8574=CARTESIAN_POINT ( 'NONE',  ( 12.34374999795161543, 3.114526743279308896, -3.846120219227901149 ) ) ;
#8618=VECTOR ( 'NONE', #16641, 1000.000000000000000 ) ;
#8662=DIRECTION ( 'NONE',  ( 0.000000000000000000, 0.000000000000000000, 1.000000000000000000 ) ) ;
#8669=CARTESIAN_POINT ( 'NONE',  ( 13.00000000000000888, -4.521642095224331470, -1.858077407906666867 ) ) ;
#8674=AXIS2_PLACEMENT_3D ( 'NONE', #2530, #16250, #17558 ) ;
#8675=B_SPLINE_CURVE_WITH_KNOTS ( 'NONE', 3,
 ( #19690, #5973, #7574, #4190, #16597, #16804, #1190, #10402, #4290, #13691 ),
 .UNSPECIFIED., .F., .F.,
 ( 4, 3, 3, 4 ),
 ( 0.000000000000000000, 0.0001875345074742622623, 0.0003808595644229699441, 0.0005744879655065562602 ),
 .UNSPECIFIED. ) ;
#8678=EDGE_CURVE ( 'NONE', #2569, #9700, #18278, .T. ) ;
#8686=AXIS2_PLACEMENT_3D ( 'NONE', #1319, #8924, #4419 ) ;
#8698=CARTESIAN_POINT ( 'NONE',  ( 11.31249999590322375, -1.185096637661254171, 5.575441324182689229 ) ) ;
#8727=ADVANCED_FACE ( 'NONE', ( #4686 ), #5635, .F. ) ;
#8739=CARTESIAN_POINT ( 'NONE',  ( -2.000000000000001776, 7.960204194457801393E-16, -6.500000000000000888 ) ) ;
#8743=DIRECTION ( 'NONE',  ( 0.000000000000000000, 0.7315216790650488354, 0.6818181818181822118 ) ) ;
#8769=EDGE_CURVE ( 'NONE', #16782, #2569, #5169, .T. ) ;
#8770=CARTESIAN_POINT ( 'NONE',  ( 6.000000000000005329, 4.936344801571289409, 2.850000000000024070 ) ) ;
#8777=ORIENTED_EDGE ( 'NONE', *, *, #7039, .T. ) ;
#8782=CARTESIAN_POINT ( 'NONE',  ( 15.31249999590322552, 3.350375938067097881, 4.611396867937200383 ) ) ;
#8793=DIRECTION ( 'NONE',  ( -1.000000000000000000, 0.000000000000000000, 0.000000000000000000 ) ) ;
#8797=EDGE_CURVE ( 'NONE', #11866, #9454, #14389, .T. ) ;
#8800=CARTESIAN_POINT ( 'NONE',  ( 10.46874999795161720, 1.016293382781477961, -4.781284448697179279 ) ) ;
#8813=EDGE_LOOP ( 'NONE', ( #3946, #4267, #320, #12559 ) ) ;
#8814=CARTESIAN_POINT ( 'NONE',  ( 13.00000000000000000, -4.333424887442987483, -2.261628166637620119 ) ) ;
#8824=CARTESIAN_POINT ( 'NONE',  ( 2.999999999999998224, 0.000000000000000000, 0.000000000000000000 ) ) ;
#8833=CYLINDRICAL_SURFACE ( 'NONE', #2422, 5.700000000000001954 ) ;
#8834=CARTESIAN_POINT ( 'NONE',  ( 12.34374999795161543, -3.114526743279282250, 3.846120219227923798 ) ) ;
#8836=ORIENTED_EDGE ( 'NONE', *, *, #2536, .T. ) ;
#8841=LINE ( 'NONE', #2823, #8618 ) ;
#8845=CARTESIAN_POINT ( 'NONE',  ( 11.96874999795161365, -1.773574444220693325, -4.620319390059841602 ) ) ;
#8853=AXIS2_PLACEMENT_3D ( 'NONE', #16524, #4610, #2799 ) ;
#8864=CARTESIAN_POINT ( 'NONE',  ( 13.00000000000000533, 4.611396867937201272, 3.350375938067096548 ) ) ;
#8882=ORIENTED_EDGE ( 'NONE', *, *, #16191, .F. ) ;
#8899=CARTESIAN_POINT ( 'NONE',  ( 14.84374999795161543, -4.861323657744410554, 0.5109457054261454800 ) ) ;
#8905=CARTESIAN_POINT ( 'NONE',  ( 10.46874999795161720, 4.648860486681953397, -1.510506337161861667 ) ) ;
#8917=PLANE ( 'NONE',  #16553 ) ;
#8924=DIRECTION ( 'NONE',  ( -1.000000000000000000, -0.000000000000000000, -0.000000000000000000 ) ) ;
#8929=CARTESIAN_POINT ( 'NONE',  ( 9.812499995903223748, 5.574407415329156734, 1.493657965219523875 ) ) ;
#8933=LINE ( 'NONE', #15036, #19479 ) ;
#8949=CARTESIAN_POINT ( 'NONE',  ( 2.999999999999998224, 3.218695387886217230, -3.000000000000000000 ) ) ;
#8976=PLANE ( 'NONE',  #3608 ) ;
#8982=( NAMED_UNIT ( * ) PLANE_ANGLE_UNIT ( ) SI_UNIT ( $, .RADIAN. ) );
#8999=CARTESIAN_POINT ( 'NONE',  ( 13.34374999795161365, -4.150607464521812062, 2.695436003842704764 ) ) ;
#9001=LINE ( 'NONE', #2786, #10892 ) ;
#9013=FACE_OUTER_BOUND ( 'NONE', #2759, .T. ) ;
#9020=CIRCLE ( 'NONE', #18911, 5.700000000000001954 ) ;
#9028=CARTESIAN_POINT ( 'NONE',  ( 10.31249999590322552, 5.207209108562820710, 2.318398865532073749 ) ) ;
#9034=FACE_OUTER_BOUND ( 'NONE', #1815, .T. ) ;
#9040=CARTESIAN_POINT ( 'NONE',  ( 13.96874999795161365, 1.280903732194486722, -4.780397808154247308 ) ) ;
#9044=MECHANICAL_DESIGN_GEOMETRIC_PRESENTATION_REPRESENTATION('',(#9681),#3598);
#9045=CYLINDRICAL_SURFACE ( 'NONE', #12190, 5.700000000000001954 ) ;
#9081=FACE_OUTER_BOUND ( 'NONE', #406, .T. ) ;
#9082=CARTESIAN_POINT ( 'NONE',  ( 13.81249999590322552, 5.142044285764750811, 2.620002426024544029 ) ) ;
#9083=DIRECTION ( 'NONE',  ( 0.000000000000000000, 0.7315216790650488354, 0.6818181818181822118 ) ) ;
#9084=EDGE_CURVE ( 'NONE', #16572, #2028, #15375, .T. ) ;
#9098=( BOUNDED_SURFACE ( )  B_SPLINE_SURFACE ( 1, 2, ( 
 ( #2211, #624, #19210, #12728, #18824, #12925, #3617, #5107, #6701, #19023, #11333, #17431, #15928, #11427, #17527, #3814, #2794 ),
 ( #18022, #7184, #18114, #7086, #16611, #16316, #5694, #5896, #1110, #13306, #5597, #10610, #12112, #11709, #4207, #15012, #4403 ) ),
 .UNSPECIFIED., .F., .F., .F. ) 
 B_SPLINE_SURFACE_WITH_KNOTS ( ( 2, 2 ),
 ( 3, 2, 2, 2, 2, 2, 2, 2, 3 ),
 ( 0.000000000000000000, 1.000000000000000000 ),
 ( 0.000000000000000000, 0.05000000000000000278, 0.1000000000000000056, 0.1499999999999999944, 0.2000000000000000111, 0.2500000000000000000, 0.2999999999999999889, 0.3499999999999999778, 0.4000000000000000222 ),
 .UNSPECIFIED. ) 
 GEOMETRIC_REPRESENTATION_ITEM ( )  RATIONAL_B_SPLINE_SURFACE ( (
 ( 1.000000000000000000, 0.9876883405951377704, 1.000000000000000000, 0.9876883405951377704, 1.000000000000000000, 0.9876883405951377704, 1.000000000000000000, 0.9876883405951377704, 1.000000000000000000, 0.9876883405951377704, 1.000000000000000000, 0.9876883405951377704, 1.000000000000000000, 0.9876883405951377704, 1.000000000000000000, 0.9876883405951377704, 1.000000000000000000),
 ( 1.000000000000000000, 0.9876883405951377704, 1.000000000000000000, 0.9876883405951377704, 1.000000000000000000, 0.9876883405951377704, 1.000000000000000000, 0.9876883405951377704, 1.000000000000000000, 0.9876883405951377704, 1.000000000000000000, 0.9876883405951377704, 1.000000000000000000, 0.9876883405951377704, 1.000000000000000000, 0.9876883405951377704, 1.000000000000000000) ) ) 
 REPRESENTATION_ITEM ( '' )  SURFACE ( )  );
#9102=CARTESIAN_POINT ( 'NONE',  ( 10.34374999795161543, -0.2590123213421313686, 4.942249507334556036 ) ) ;
#9105=CARTESIAN_POINT ( 'NONE',  ( 7.312499995903225525, -4.936344801571327601, 2.849999999999954348 ) ) ;
#9107=CARTESIAN_POINT ( 'NONE',  ( 7.000000000000005329, 5.575441324182695446, -1.185096637661215091 ) ) ;
#9114=CARTESIAN_POINT ( 'NONE',  ( 14.46874999795161720, -4.861323657744410554, 0.5109457054261454800 ) ) ;
#9116=CARTESIAN_POINT ( 'NONE',  ( 14.84374999795161543, 2.873153789725825913, 3.954556930911861112 ) ) ;
#9124=VERTEX_POINT ( 'NONE', #4467 ) ;
#9130=CARTESIAN_POINT ( 'NONE',  ( 7.812499995903224637, 5.387740456496233676, -2.068159791354184041 ) ) ;
#9143=CYLINDRICAL_SURFACE ( 'NONE', #9455, 5.700000000000001954 ) ;
#9152=CARTESIAN_POINT ( 'NONE',  ( 13.00000000000000000, 3.840809689103004576, -4.211671987713725862 ) ) ;
#9162=FACE_OUTER_BOUND ( 'NONE', #14067, .T. ) ;
#9179=CARTESIAN_POINT ( 'NONE',  ( 13.00000000000000000, -0.2705398332808414130, -4.881009025374877908 ) ) ;
#9184=( NAMED_UNIT ( * ) PLANE_ANGLE_UNIT ( ) SI_UNIT ( $, .RADIAN. ) );
#9203=CARTESIAN_POINT ( 'NONE',  ( 7.078124996927420476, 4.584782303107579615, 2.647025296875021638 ) ) ;
#9216=CARTESIAN_POINT ( 'NONE',  ( 8.500000000000007105, 5.574407415329156734, 1.493657965219523875 ) ) ;
#9222=CARTESIAN_POINT ( 'NONE',  ( 10.46874999795161720, -4.648860486681964055, 1.510506337161829027 ) ) ;
#9234=CARTESIAN_POINT ( 'NONE',  ( 13.00000000000000178, 7.960204194457801393E-16, -6.500000000000002665 ) ) ;
#9235=EDGE_LOOP ( 'NONE', ( #4697, #2650, #7301, #3932 ) ) ;
#9237=DIRECTION ( 'NONE',  ( -1.000000000000000000, -0.000000000000000000, -0.000000000000000000 ) ) ;
#9244=DIRECTION ( 'NONE',  ( 0.000000000000000000, 0.000000000000000000, 1.000000000000000000 ) ) ;
#9251=ORIENTED_EDGE ( 'NONE', *, *, #8365, .T. ) ;
#9253=LINE ( 'NONE', #7836, #11167 ) ;
#9258=ORIENTED_EDGE ( 'NONE', *, *, #9370, .F. ) ;
#9267=CARTESIAN_POINT ( 'NONE',  ( 8.843749997951615427, 2.873153789725825469, -3.954556930911862000 ) ) ;
#9272=VERTEX_POINT ( 'NONE', #11651 ) ;
#9295=CARTESIAN_POINT ( 'NONE',  ( 7.500000000000005329, -3.143139765844555900, -4.840010801796527318 ) ) ;
#9299=PLANE ( 'NONE',  #15737 ) ;
#9316=CARTESIAN_POINT ( 'NONE',  ( -0.000000000000000000, 0.000000000000000000, 0.000000000000000000 ) ) ;
#9318=CARTESIAN_POINT ( 'NONE',  ( 11.34374999795161543, -4.888101187500005551, 0.7741991708318548548 ) ) ;
#9343=VERTEX_POINT ( 'NONE', #7631 ) ;
#9348=DIRECTION ( 'NONE',  ( -0.4999999999999980016, -0.7500000000000048850, 0.4330127018922129700 ) ) ;
#9362=CARTESIAN_POINT ( 'NONE',  ( 8.343749997951611874, 4.942249507334556924, -0.2590123213420971182 ) ) ;
#9368=CARTESIAN_POINT ( 'NONE',  ( 6.843749997951615427, 0.000000000000000000, -4.888101187500000222 ) ) ;
#9370=EDGE_CURVE ( 'NONE', #2028, #5529, #12941, .T. ) ;
#9374=ORIENTED_EDGE ( 'NONE', *, *, #174, .F. ) ;
#9377=CARTESIAN_POINT ( 'NONE',  ( 12.96874999795161543, -0.2590123213420631454, -4.942249507334558700 ) ) ;
#9379=CARTESIAN_POINT ( 'NONE',  ( 13.00000000000000178, -0.4594918047638649194, -4.866883308198429958 ) ) ;
#9382=EDGE_CURVE ( 'NONE', #18748, #15548, #800, .T. ) ;
#9383=CARTESIAN_POINT ( 'NONE',  ( -2.000000000000001776, 0.000000000000000000, 4.400000000000000355 ) ) ;
#9395=DIRECTION ( 'NONE',  ( 0.000000000000000000, 0.000000000000000000, 1.000000000000000000 ) ) ;
#9396=CARTESIAN_POINT ( 'NONE',  ( 10.34374999795161543, -4.409619785863921670, 2.246813503491803310 ) ) ;
#9407=ORIENTED_EDGE ( 'NONE', *, *, #8797, .T. ) ;
#9408=CARTESIAN_POINT ( 'NONE',  ( 13.46874999795161543, 3.954556930911862000, 2.873153789725825025 ) ) ;
#9412=LINE ( 'NONE', #103, #3113 ) ;
#9415=CARTESIAN_POINT ( 'NONE',  ( 10.46874999795161720, 3.632567103900523620, 3.270778111535338262 ) ) ;
#9423=CARTESIAN_POINT ( 'NONE',  ( 8.000000000000005329, -2.318398865532001363, -5.207209108562852684 ) ) ;
#9449=EDGE_CURVE ( 'NONE', #720, #15404, #2385, .T. ) ;
#9454=VERTEX_POINT ( 'NONE', #11603 ) ;
#9455=AXIS2_PLACEMENT_3D ( 'NONE', #15248, #1630, #10936 ) ;
#9456=CARTESIAN_POINT ( 'NONE',  ( 9.000000000000005329, -5.207209108562803834, -2.318398865532109721 ) ) ;
#9463=PRODUCT_CONTEXT ( 'NONE', #1638, 'mechanical' ) ;
#9465=CARTESIAN_POINT ( 'NONE',  ( 7.968749997951616315, 4.942249507334556924, -0.2590123213420971182 ) ) ;
#9480=AXIS2_PLACEMENT_3D ( 'NONE', #2184, #6774, #3685 ) ;
#9484=DIRECTION ( 'NONE',  ( -0.4999999999999979461, 0.000000000000000000, -0.8660254037844398178 ) ) ;
#9485=VECTOR ( 'NONE', #17388, 1000.000000000000227 ) ;
#9496=CARTESIAN_POINT ( 'NONE',  ( 12.84374999795161543, -4.648860486681943627, -1.510506337161893642 ) ) ;
#9499=CARTESIAN_POINT ( 'NONE',  ( 12.96874999795161543, 4.150607464521828938, -2.695436003842674566 ) ) ;
#9530=FACE_OUTER_BOUND ( 'NONE', #4689, .T. ) ;
#9531=DIRECTION ( 'NONE',  ( -0.4999999999999979461, 0.000000000000000000, 0.8660254037844398178 ) ) ;
#9536=ORIENTED_EDGE ( 'NONE', *, *, #4191, .T. ) ;
#9556=CARTESIAN_POINT ( 'NONE',  ( 12.81249999590322552, 3.631840208645857437, -4.484949146646330931 ) ) ;
#9571=ADVANCED_FACE ( 'NONE', ( #14710 ), #8212, .F. ) ;
#9584=AXIS2_PLACEMENT_3D ( 'NONE', #12068, #1359, #4657 ) ;
#9589=CARTESIAN_POINT ( 'NONE',  ( 13.46874999795161543, 4.465502636338051445, -1.988169868018530906 ) ) ;
#9592=CARTESIAN_POINT ( 'NONE',  ( 6.500000000000005329, -4.484949146646330931, -3.631840208645857437 ) ) ;
#9597=ADVANCED_FACE ( 'NONE', ( #5684 ), #156, .F. ) ;
#9599=DIRECTION ( 'NONE',  ( 0.000000000000000000, -0.6818181818181815457, -0.7315216790650493905 ) ) ;
#9603=CARTESIAN_POINT ( 'NONE',  ( 13.50000000000000533, 4.080749450109650844, 4.080749450109649956 ) ) ;
#9609=CARTESIAN_POINT ( 'NONE',  ( 6.000000000000005329, 4.936344801571308061, -2.849999999999988987 ) ) ;
#9626=( BOUNDED_SURFACE ( )  B_SPLINE_SURFACE ( 1, 2, ( 
 ( #19005, #5192, #15909, #3695, #2292, #3795, #6681, #2389, #12906, #11500, #8297, #5296, #6878, #9815, #804, #18902, #11403 ),
 ( #9916, #8405, #14515, #16111, #16002, #14408, #13006, #8503, #17601, #19097, #606, #15477, #11068, #9377, #668, #15573, #15671 ) ),
 .UNSPECIFIED., .F., .F., .F. ) 
 B_SPLINE_SURFACE_WITH_KNOTS ( ( 2, 2 ),
 ( 3, 2, 2, 2, 2, 2, 2, 2, 3 ),
 ( 0.000000000000000000, 1.000000000000000000 ),
 ( 0.000000000000000000, 0.05000000000000000278, 0.1000000000000000056, 0.1499999999999999944, 0.2000000000000000111, 0.2500000000000000000, 0.2999999999999999889, 0.3499999999999999778, 0.4000000000000000222 ),
 .UNSPECIFIED. ) 
 GEOMETRIC_REPRESENTATION_ITEM ( )  RATIONAL_B_SPLINE_SURFACE ( (
 ( 1.000000000000000000, 0.9876883405951377704, 1.000000000000000000, 0.9876883405951377704, 1.000000000000000000, 0.9876883405951377704, 1.000000000000000000, 0.9876883405951377704, 1.000000000000000000, 0.9876883405951377704, 1.000000000000000000, 0.9876883405951377704, 1.000000000000000000, 0.9876883405951377704, 1.000000000000000000, 0.9876883405951377704, 1.000000000000000000),
 ( 1.000000000000000000, 0.9876883405951377704, 1.000000000000000000, 0.9876883405951377704, 1.000000000000000000, 0.9876883405951377704, 1.000000000000000000, 0.9876883405951377704, 1.000000000000000000, 0.9876883405951377704, 1.000000000000000000, 0.9876883405951377704, 1.000000000000000000, 0.9876883405951377704, 1.000000000000000000, 0.9876883405951377704, 1.000000000000000000) ) ) 
 REPRESENTATION_ITEM ( '' )  SURFACE ( )  );
#9643=ORIENTED_EDGE ( 'NONE', *, *, #17258, .T. ) ;
#9655=DIRECTION ( 'NONE',  ( -0.4999999999999977240, 0.7499999999999961142, 0.4330127018922284576 ) ) ;
#9656=CARTESIAN_POINT ( 'NONE',  ( 14.84374999795161543, 4.861323657744413218, -0.5109457054261112852 ) ) ;
#9681=STYLED_ITEM ( 'NONE', ( #3966 ), #2634 ) ;
#9700=VERTEX_POINT ( 'NONE', #12197 ) ;
#9724=DIRECTION ( 'NONE',  ( -1.000000000000000000, 0.000000000000000000, 0.000000000000000000 ) ) ;
#9727=CARTESIAN_POINT ( 'NONE',  ( 13.31249999590322730, -5.421022142882365280, -1.761396867937238042 ) ) ;
#9732=CARTESIAN_POINT ( 'NONE',  ( 13.00000000000000178, 4.568735188514060575, 1.737869959597756697 ) ) ;
#9761=CARTESIAN_POINT ( 'NONE',  ( 14.81249999590322552, 5.574407415329178939, -1.493657965219446382 ) ) ;
#9762=CARTESIAN_POINT ( 'NONE',  ( 2.999999999999998224, -3.950217066951267064, 3.681818181818180769 ) ) ;
#9766=EDGE_LOOP ( 'NONE', ( #16634, #6594, #2971, #5999 ) ) ;
#9768=CARTESIAN_POINT ( 'NONE',  ( 12.84374999795161543, -3.632567103900546712, 3.270778111535314281 ) ) ;
#9775=CARTESIAN_POINT ( 'NONE',  ( 6.468749997951615427, 4.233219804643887585, -2.444050593749990341 ) ) ;
#9783=CARTESIAN_POINT ( 'NONE',  ( 8.500000000000005329, -4.080749450109678378, 4.080749450109622423 ) ) ;
#9790=ORIENTED_EDGE ( 'NONE', *, *, #18465, .F. ) ;
#9796=ORIENTED_EDGE ( 'NONE', *, *, #15421, .T. ) ;
#9797=CARTESIAN_POINT ( 'NONE',  ( 11.46874999795161543, 2.444050593750049405, -4.233219804643852946 ) ) ;
#9798=CARTESIAN_POINT ( 'NONE',  ( 13.00000000000000178, -3.908719486245979091, 2.935207862670018653 ) ) ;
#9810=ORIENTED_EDGE ( 'NONE', *, *, #14618, .F. ) ;
#9815=CARTESIAN_POINT ( 'NONE',  ( 13.34374999795161365, -0.2590123213420631454, -4.942249507334558700 ) ) ;
#9823=CARTESIAN_POINT ( 'NONE',  ( 10.31249999590322552, -4.611396867937225252, 3.350375938067065462 ) ) ;
#9833=DIRECTION ( 'NONE',  ( 0.000000000000000000, 0.000000000000000000, 1.000000000000000000 ) ) ;
#9841=CARTESIAN_POINT ( 'NONE',  ( 13.00000000000000178, 0.000000000000000000, 0.000000000000000000 ) ) ;
#9847=EDGE_CURVE ( 'NONE', #15, #13643, #5278, .T. ) ;
#9875=DIRECTION ( 'NONE',  ( -1.000000000000000000, 0.000000000000000000, 0.000000000000000000 ) ) ;
#9889=ORIENTED_EDGE ( 'NONE', *, *, #6366, .T. ) ;
#9893=CARTESIAN_POINT ( 'NONE',  ( 13.00000000000000178, 3.789407127742559833, -3.087705756618140285 ) ) ;
#9906=CARTESIAN_POINT ( 'NONE',  ( 10.34374999795161543, 4.150607464521792522, 2.695436003842732298 ) ) ;
#9913=CARTESIAN_POINT ( 'NONE',  ( 11.81249999590322552, 3.631840208645794821, 4.484949146646379781 ) ) ;
#9916=CARTESIAN_POINT ( 'NONE',  ( 6.468749997951615427, -4.233219804643904460, 2.444050593749960587 ) ) ;
#9920=CARTESIAN_POINT ( 'NONE',  ( 9.312499995903225525, -3.350375938067129855, 4.611396867937178179 ) ) ;
#9925=ORIENTED_EDGE ( 'NONE', *, *, #6341, .T. ) ;
#9959=ORIENTED_EDGE ( 'NONE', *, *, #14486, .F. ) ;
#9966=LINE ( 'NONE', #19151, #15307 ) ;
#9967=CARTESIAN_POINT ( 'NONE',  ( 7.312499995903225525, -3.980288726281172656E-14, 5.700000000000001066 ) ) ;
#9977=CARTESIAN_POINT ( 'NONE',  ( 12.50000000000000533, -5.142044285764733935, -2.620002426024580000 ) ) ;
#9979=CARTESIAN_POINT ( 'NONE',  ( 6.968749997951614539, -4.620319390059842490, 1.773574444220693103 ) ) ;
#9985=CARTESIAN_POINT ( 'NONE',  ( 13.00000000000000533, -5.207209108562836697, 2.318398865532038666 ) ) ;
#9987=CIRCLE ( 'NONE', #3902, 40.00000000000000711 ) ;
#9989=VECTOR ( 'NONE', #19764, 1000.000000000000000 ) ;
#9991=CARTESIAN_POINT ( 'NONE',  ( 11.96874999795161365, 3.114526743279308896, -3.846120219227901593 ) ) ;
#9993=CARTESIAN_POINT ( 'NONE',  ( 10.31249999590322552, -0.5958122406255588199, -5.668774803599165857 ) ) ;
#10007=CARTESIAN_POINT ( 'NONE',  ( 12.31249999590322552, 2.849999999999989875, 4.936344801571308061 ) ) ;
#10009=VECTOR ( 'NONE', #9348, 1000.000000000000114 ) ;
#10019=CARTESIAN_POINT ( 'NONE',  ( 13.34374999795161365, -4.409619785863891472, -2.246813503491864150 ) ) ;
#10033=VERTEX_POINT ( 'NONE', #17657 ) ;
#10034=DIRECTION ( 'NONE',  ( -1.000000000000000000, 0.000000000000000000, 0.000000000000000000 ) ) ;
#10038=CARTESIAN_POINT ( 'NONE',  ( 13.00000000000000178, -3.789407127742538517, 3.087705756618167374 ) ) ;
#10042=EDGE_CURVE ( 'NONE', #1853, #12828, #2709, .T. ) ;
#10061=CARTESIAN_POINT ( 'NONE',  ( -2.000000000000001776, 3.478305785123969152, -3.241971077674649315 ) ) ;
#10065=EDGE_CURVE ( 'NONE', #11016, #18417, #11358, .T. ) ;
#10080=EDGE_CURVE ( 'NONE', #9454, #2779, #3481, .T. ) ;
#10082=ORIENTED_EDGE ( 'NONE', *, *, #5985, .F. ) ;
#10084=CARTESIAN_POINT ( 'NONE',  ( 13.46874999795161543, -4.465502636338038123, 1.988169868018562880 ) ) ;
#10086=DIRECTION ( 'NONE',  ( 0.000000000000000000, 0.000000000000000000, 1.000000000000000000 ) ) ;
#10090=CARTESIAN_POINT ( 'NONE',  ( 13.00000000000000533, -3.985098679772345331, 2.831373229855499662 ) ) ;
#10096=CARTESIAN_POINT ( 'NONE',  ( 7.343749997951615427, -4.620319390059842490, 1.773574444220693103 ) ) ;
#10101=EDGE_LOOP ( 'NONE', ( #13718, #2974, #148, #3654, #5065 ) ) ;
#10102=CARTESIAN_POINT ( 'NONE',  ( 9.812499995903225525, 5.574407415329157622, 1.493657965219523875 ) ) ;
#10124=CARTESIAN_POINT ( 'NONE',  ( 11.81249999590322552, -3.631840208645763735, -4.484949146646406426 ) ) ;
#10133=ORIENTED_EDGE ( 'NONE', *, *, #6340, .T. ) ;
#10144=CARTESIAN_POINT ( 'NONE',  ( 7.468749997951615427, 1.510506337161861445, -4.648860486681953397 ) ) ;
#10155=CARTESIAN_POINT ( 'NONE',  ( 6.000000000000005329, 4.936344801571289409, 2.850000000000024070 ) ) ;
#10161=ADVANCED_FACE ( 'NONE', ( #16749 ), #19190, .F. ) ;
#10176=CARTESIAN_POINT ( 'NONE',  ( 7.500000000000005329, 3.143139765844590983, 4.840010801796506890 ) ) ;
#10182=CARTESIAN_POINT ( 'NONE',  ( 10.84374999795161543, 1.016293382781477961, -4.781284448697179279 ) ) ;
#10183=EDGE_LOOP ( 'NONE', ( #3414, #18475, #2555, #3644 ) ) ;
#10188=CARTESIAN_POINT ( 'NONE',  ( 8.843749997951615427, -4.861323657744403448, -0.5109457054262123155 ) ) ;
#10202=LINE ( 'NONE', #7265, #18293 ) ;
#10210=CARTESIAN_POINT ( 'NONE',  ( 7.468749997951615427, -3.270778111535287191, -3.632567103900569361 ) ) ;
#10211=ADVANCED_FACE ( 'NONE', ( #11035 ), #9143, .F. ) ;
#10214=DIRECTION ( 'NONE',  ( 1.000000000000000000, 0.000000000000000000, 0.000000000000000000 ) ) ;
#10222=LINE ( 'NONE', #19308, #5972 ) ;
#10233=CARTESIAN_POINT ( 'NONE',  ( 2.999999999999998224, -3.218695387886215009, -3.000000000000001776 ) ) ;
#10243=FACE_OUTER_BOUND ( 'NONE', #7841, .T. ) ;
#10245=CARTESIAN_POINT ( 'NONE',  ( 11.34374999795161543, -1.773574444220757496, 4.620319390059819398 ) ) ;
#10251=CARTESIAN_POINT ( 'NONE',  ( 7.468749997951615427, 3.270778111535313837, 3.632567103900546712 ) ) ;
#10255=CARTESIAN_POINT ( 'NONE',  ( 8.468749997951615427, -4.861323657744403448, -0.5109457054262123155 ) ) ;
#10258=VECTOR ( 'NONE', #11801, 1000.000000000000114 ) ;
#10280=ORIENTED_EDGE ( 'NONE', *, *, #12220, .T. ) ;
#10286=ORIENTED_EDGE ( 'NONE', *, *, #15814, .F. ) ;
#10302=LINE ( 'NONE', #16401, #13052 ) ;
#10310=CARTESIAN_POINT ( 'NONE',  ( 13.81249999590322552, -4.840010801796506890, 3.143139765844590983 ) ) ;
#10311=CARTESIAN_POINT ( 'NONE',  ( 11.81249999590322552, -3.631840208645764179, -4.484949146646406426 ) ) ;
#10329=CARTESIAN_POINT ( 'NONE',  ( 11.34374999795161543, 4.888101187500000222, -0.7741991708318890497 ) ) ;
#10338=AXIS2_PLACEMENT_3D ( 'NONE', #16343, #12115, #16824 ) ;
#10355=CARTESIAN_POINT ( 'NONE',  ( 11.00000000000000711, -2.849999999999954792, -4.936344801571327601 ) ) ;
#10381=ORIENTED_EDGE ( 'NONE', *, *, #979, .T. ) ;
#10387=( BOUNDED_SURFACE ( )  B_SPLINE_SURFACE ( 1, 2, ( 
 ( #7098, #4615, #17215, #11012, #12222, #7, #6100, #13918, #10721, #9318, #18323, #7900, #407, #6488, #12518, #12619, #213 ),
 ( #16832, #18515, #3110, #16927, #18705, #13816, #15326, #1611, #9222, #14015, #1809, #7701, #5006, #3506, #15617, #3206, #14110 ) ),
 .UNSPECIFIED., .F., .F., .F. ) 
 B_SPLINE_SURFACE_WITH_KNOTS ( ( 2, 2 ),
 ( 3, 2, 2, 2, 2, 2, 2, 2, 3 ),
 ( 0.000000000000000000, 1.000000000000000000 ),
 ( 0.000000000000000000, 0.05000000000000000278, 0.1000000000000000056, 0.1499999999999999944, 0.2000000000000000111, 0.2500000000000000000, 0.2999999999999999889, 0.3499999999999999778, 0.4000000000000000222 ),
 .UNSPECIFIED. ) 
 GEOMETRIC_REPRESENTATION_ITEM ( )  RATIONAL_B_SPLINE_SURFACE ( (
 ( 1.000000000000000000, 0.9876883405951377704, 1.000000000000000000, 0.9876883405951377704, 1.000000000000000000, 0.9876883405951377704, 1.000000000000000000, 0.9876883405951377704, 1.000000000000000000, 0.9876883405951377704, 1.000000000000000000, 0.9876883405951377704, 1.000000000000000000, 0.9876883405951377704, 1.000000000000000000, 0.9876883405951377704, 1.000000000000000000),
 ( 1.000000000000000000, 0.9876883405951377704, 1.000000000000000000, 0.9876883405951377704, 1.000000000000000000, 0.9876883405951377704, 1.000000000000000000, 0.9876883405951377704, 1.000000000000000000, 0.9876883405951377704, 1.000000000000000000, 0.9876883405951377704, 1.000000000000000000, 0.9876883405951377704, 1.000000000000000000, 0.9876883405951377704, 1.000000000000000000) ) ) 
 REPRESENTATION_ITEM ( '' )  SURFACE ( )  );
#10390=CARTESIAN_POINT ( 'NONE',  ( 8.843749997951615427, 2.873153789725825469, -3.954556930911862000 ) ) ;
#10402=CARTESIAN_POINT ( 'NONE',  ( 12.99999999999999467, 4.521642095224343905, 1.858077407906634892 ) ) ;
#10408=CARTESIAN_POINT ( 'NONE',  ( 14.81249999590322552, 1.493657965219562067, -5.574407415329146964 ) ) ;
#10414=CARTESIAN_POINT ( 'NONE',  ( 7.968749997951616315, 2.246813503491833508, -4.409619785863906571 ) ) ;
#10419=ORIENTED_EDGE ( 'NONE', *, *, #5009, .T. ) ;
#10421=CYLINDRICAL_SURFACE ( 'NONE', #14723, 5.700000000000001954 ) ;
#10422=CARTESIAN_POINT ( 'NONE',  ( 13.46874999795161543, 3.954556930911862000, 2.873153789725825025 ) ) ;
#10423=CARTESIAN_POINT ( 'NONE',  ( 13.00000000000000533, 0.5958122406256767256, -5.668774803599153422 ) ) ;
#10438=DIRECTION ( 'NONE',  ( -1.000000000000000000, 0.000000000000000000, 0.000000000000000000 ) ) ;
#10446=CARTESIAN_POINT ( 'NONE',  ( 13.00000000000000178, 4.568735188514060575, 1.737869959597756697 ) ) ;
#10449=ADVANCED_FACE ( 'NONE', ( #6328 ), #6271, .F. ) ;
#10464=CARTESIAN_POINT ( 'NONE',  ( 7.968749997951616315, -4.942249507334558700, 0.2590123213420630899 ) ) ;
#10471=ORIENTED_EDGE ( 'NONE', *, *, #13974, .T. ) ;
#10473=APPLICATION_CONTEXT ( 'automotive_design' ) ;
#10497=AXIS2_PLACEMENT_3D ( 'NONE', #17581, #17777, #10086 ) ;
#10498=DIRECTION ( 'NONE',  ( 1.000000000000000000, 0.000000000000000000, 0.000000000000000000 ) ) ;
#10505=ADVANCED_FACE ( 'NONE', ( #16154, #12847 ), #11733, .T. ) ;
#10516=CARTESIAN_POINT ( 'NONE',  ( 7.968749997951616315, -2.246813503491864150, 4.409619785863891472 ) ) ;
#10526=ORIENTED_EDGE ( 'NONE', *, *, #13974, .F. ) ;
#10543=CARTESIAN_POINT ( 'NONE',  ( 7.468749997951615427, -4.781284448697200595, 1.016293382781377819 ) ) ;
#10555=CARTESIAN_POINT ( 'NONE',  ( 6.000000000000005329, 0.000000000000000000, 0.000000000000000000 ) ) ;
#10557=LINE ( 'NONE', #6036, #12492 ) ;
#10562=CARTESIAN_POINT ( 'NONE',  ( 8.968749997951613651, -4.780397808154247308, -1.280903732194487166 ) ) ;
#10572=ADVANCED_FACE ( 'NONE', ( #10243 ), #18556, .F. ) ;
#10582=FACE_OUTER_BOUND ( 'NONE', #19354, .T. ) ;
#10599=CARTESIAN_POINT ( 'NONE',  ( 8.312499995903225525, 3.814044456245473835, 4.235925505221166176 ) ) ;
#10604=ORIENTED_EDGE ( 'NONE', *, *, #7750, .F. ) ;
#10610=CARTESIAN_POINT ( 'NONE',  ( 11.50000000000000355, -5.699999999999994849, -0.9027913098498961952 ) ) ;
#10617=CARTESIAN_POINT ( 'NONE',  ( 10.84374999795161543, 4.648860486681953397, -1.510506337161861667 ) ) ;
#10620=ORIENTED_EDGE ( 'NONE', *, *, #15421, .F. ) ;
#10630=VERTEX_POINT ( 'NONE', #16440 ) ;
#10632=CARTESIAN_POINT ( 'NONE',  ( 8.343749997951611874, 4.942249507334556924, -0.2590123213420975623 ) ) ;
#10640=ADVANCED_FACE ( 'NONE', ( #2716 ), #8833, .F. ) ;
#10646=CARTESIAN_POINT ( 'NONE',  ( 8.468749997951615427, 4.861323657744407001, 0.5109457054261784537 ) ) ;
#10656=DIRECTION ( 'NONE',  ( 0.000000000000000000, 0.000000000000000000, -1.000000000000000000 ) ) ;
#10665=LINE ( 'NONE', #18364, #19156 ) ;
#10675=CARTESIAN_POINT ( 'NONE',  ( -2.000000000000001776, -3.218695387886217674, 2.999999999999999112 ) ) ;
#10681=CARTESIAN_POINT ( 'NONE',  ( 11.84374999795161365, 4.888101187500000222, -2.993098736590125853E-16 ) ) ;
#10698=CARTESIAN_POINT ( 'NONE',  ( 13.00000000000000533, -0.5958122406256377568, 5.668774803599156975 ) ) ;
#10700=CARTESIAN_POINT ( 'NONE',  ( 9.500000000000003553, 0.3020334839683282979, -5.763142191869152775 ) ) ;
#10703=DIRECTION ( 'NONE',  ( 0.000000000000000000, 0.000000000000000000, 1.000000000000000000 ) ) ;
#10704=DIRECTION ( 'NONE',  ( -1.000000000000000000, -0.000000000000000000, -0.000000000000000000 ) ) ;
#10707=CARTESIAN_POINT ( 'NONE',  ( 6.000000000000005329, 0.000000000000000000, -5.700000000000001066 ) ) ;
#10714=CARTESIAN_POINT ( 'NONE',  ( 7.500000000000005329, 5.763142191869157216, -0.3020334839682475847 ) ) ;
#10721=CARTESIAN_POINT ( 'NONE',  ( 10.84374999795161543, -4.648860486681964055, 1.510506337161829027 ) ) ;
#10748=CARTESIAN_POINT ( 'NONE',  ( 6.234374998975811266, -4.584782303107616031, 2.647025296874957689 ) ) ;
#10776=CARTESIAN_POINT ( 'NONE',  ( -2.000000000000001776, -3.950217066951263956, -3.681818181818183877 ) ) ;
#10791=CARTESIAN_POINT ( 'NONE',  ( 6.843749997951615427, -4.233219804643852946, -2.444050593750049849 ) ) ;
#10794=CARTESIAN_POINT ( 'NONE',  ( 11.50000000000000355, 3.631840208645857437, -4.484949146646330931 ) ) ;
#10795=ADVANCED_FACE ( 'NONE', ( #9530 ), #418, .T. ) ;
#10798=CARTESIAN_POINT ( 'NONE',  ( -2.000000000000001776, 3.950217066951266176, -3.681818181818181213 ) ) ;
#10802=CARTESIAN_POINT ( 'NONE',  ( 13.96874999795161365, 3.499494075959816541, 3.499494075959815653 ) ) ;
#10811=CARTESIAN_POINT ( 'NONE',  ( 13.00000000000000533, -0.5958122406256377568, 5.668774803599156975 ) ) ;
#10813=ORIENTED_EDGE ( 'NONE', *, *, #4065, .F. ) ;
#10839=CARTESIAN_POINT ( 'NONE',  ( 13.00000000000000000, 0.2080849974989116558, 4.883670121236158401 ) ) ;
#10851=CIRCLE ( 'NONE', #18208, 5.700000000000001954 ) ;
#10853=CARTESIAN_POINT ( 'NONE',  ( 7.812499995903224637, -4.484949146646330931, -3.631840208645857437 ) ) ;
#10859=DIRECTION ( 'NONE',  ( 0.000000000000000000, 0.000000000000000000, 1.000000000000000000 ) ) ;
#10881=ORIENTED_EDGE ( 'NONE', *, *, #18771, .T. ) ;
#10892=VECTOR ( 'NONE', #18302, 1000.000000000000000 ) ;
#10894=CARTESIAN_POINT ( 'NONE',  ( 7.000000000000005329, -3.814044456245443193, -4.235925505221191933 ) ) ;
#10904=( BOUNDED_CURVE ( )  B_SPLINE_CURVE ( 2, ( #299, #12610, #4995, #8500, #17597, #10102, #16202, #2384, #2476, #9913, #10007, #6677, #8398 ),
 .UNSPECIFIED., .F., .F. ) 
 B_SPLINE_CURVE_WITH_KNOTS ( ( 3, 2, 2, 2, 2, 2, 3 ),
 ( 0.000000000000000000, 0.05000000000000000278, 0.1000000000000000056, 0.1499999999999999944, 0.2000000000000000111, 0.2500000000000000000, 0.2843253191101273170 ),
 .UNSPECIFIED. ) 
 CURVE ( )  GEOMETRIC_REPRESENTATION_ITEM ( )  RATIONAL_B_SPLINE_CURVE ( ( 1.000000000000000000, 0.9876883405951377704, 1.000000000000000000, 0.9876883405951377704, 1.000000000000000000, 0.9876883405951377704, 1.000000000000000000, 0.9876883405951377704, 1.000000000000000000, 0.9876883405951377704, 1.000000000000000000, 0.9915479672430580482, 0.9947006833465674713 ) ) 
 REPRESENTATION_ITEM ( '' )  );
#10910=CARTESIAN_POINT ( 'NONE',  ( 13.00000000000000178, -3.849641071994423402, 3.458892414715191599 ) ) ;
#10914=DIRECTION ( 'NONE',  ( 0.000000000000000000, 0.000000000000000000, 1.000000000000000000 ) ) ;
#10916=CARTESIAN_POINT ( 'NONE',  ( 6.000000000000005329, -4.936344801571268093, -2.850000000000058265 ) ) ;
#10918=ORIENTED_EDGE ( 'NONE', *, *, #4191, .F. ) ;
#10936=DIRECTION ( 'NONE',  ( 0.000000000000000000, 0.000000000000000000, 1.000000000000000000 ) ) ;
#10952=CARTESIAN_POINT ( 'NONE',  ( 9.843749997951615427, -0.5109457054261099529, -4.861323657744413218 ) ) ;
#10960=CARTESIAN_POINT ( 'NONE',  ( 11.84374999795161365, 2.444050593749990785, 4.233219804643887585 ) ) ;
#10989=CARTESIAN_POINT ( 'NONE',  ( 8.843749997951615427, -2.873153789725853002, 3.954556930911842016 ) ) ;
#10992=CARTESIAN_POINT ( 'NONE',  ( 14.46874999795161720, 4.861323657744413218, -0.5109457054261112852 ) ) ;
#10993=CARTESIAN_POINT ( 'NONE',  ( 12.84374999795161543, -1.016293382781378485, -4.781284448697201483 ) ) ;
#11005=CARTESIAN_POINT ( 'NONE',  ( 6.468749997951615427, -4.233219804643852946, -2.444050593750049849 ) ) ;
#11012=CARTESIAN_POINT ( 'NONE',  ( 8.343749997951611874, -2.246813503491864150, 4.409619785863891472 ) ) ;
#11016=VERTEX_POINT ( 'NONE', #13606 ) ;
#11035=FACE_OUTER_BOUND ( 'NONE', #10101, .T. ) ;
#11048=CARTESIAN_POINT ( 'NONE',  ( 8.812499995903225525, -3.143139765844555900, -4.840010801796527318 ) ) ;
#11056=ADVANCED_FACE ( 'NONE', ( #4302 ), #13069, .F. ) ;
#11068=CARTESIAN_POINT ( 'NONE',  ( 12.46874999795161543, -1.016293382781378485, -4.781284448697201483 ) ) ;
#11072=ORIENTED_EDGE ( 'NONE', *, *, #11189, .T. ) ;
#11075=CARTESIAN_POINT ( 'NONE',  ( 6.000000000000005329, -4.936344801571268093, -2.850000000000058265 ) ) ;
#11076=AXIS2_PLACEMENT_3D ( 'NONE', #18783, #588, #5074 ) ;
#11077=EDGE_CURVE ( 'NONE', #17840, #720, #12501, .T. ) ;
#11097=CARTESIAN_POINT ( 'NONE',  ( 10.00000000000000533, 5.421022142882375938, -1.761396867937200739 ) ) ;
#11104=CARTESIAN_POINT ( 'NONE',  ( 9.968749997951617203, 4.150607464521791634, 2.695436003842732298 ) ) ;
#11120=CARTESIAN_POINT ( 'NONE',  ( 9.668198987696284163, -0.5990941410143687529, 5.700000000000001954 ) ) ;
#11132=ORIENTED_EDGE ( 'NONE', *, *, #6233, .T. ) ;
#11150=CARTESIAN_POINT ( 'NONE',  ( 11.00000000000000711, -2.849999999999954792, -4.936344801571327601 ) ) ;
#11151=CARTESIAN_POINT ( 'NONE',  ( 6.843749997951615427, -4.233219804643852946, -2.444050593750049849 ) ) ;
#11159=CARTESIAN_POINT ( 'NONE',  ( 10.34374999795161543, 4.150607464521791634, 2.695436003842732298 ) ) ;
#11167=VECTOR ( 'NONE', #3537, 1000.000000000000000 ) ;
#11184=EDGE_LOOP ( 'NONE', ( #12386, #11883, #18663, #4823 ) ) ;
#11185=CARTESIAN_POINT ( 'NONE',  ( 6.234374998975811266, -4.584782303107560963, -2.647025296875054057 ) ) ;
#11189=EDGE_CURVE ( 'NONE', #4538, #6183, #1442, .T. ) ;
#11216=CARTESIAN_POINT ( 'NONE',  ( 12.50000000000000533, -4.840010801796506001, 3.143139765844590983 ) ) ;
#11234=DIRECTION ( 'NONE',  ( -1.000000000000000000, -0.000000000000000000, -0.000000000000000000 ) ) ;
#11239=EDGE_CURVE ( 'NONE', #16572, #11644, #6900, .T. ) ;
#11246=CARTESIAN_POINT ( 'NONE',  ( 10.84374999795161543, -1.016293382781444654, 4.781284448697187273 ) ) ;
#11253=CARTESIAN_POINT ( 'NONE',  ( 10.84374999795161543, -1.016293382781444654, 4.781284448697187273 ) ) ;
#11277=DIRECTION ( 'NONE',  ( 0.000000000000000000, 0.000000000000000000, 1.000000000000000000 ) ) ;
#11298=CARTESIAN_POINT ( 'NONE',  ( 2.999999999999998224, -2.487173708821168283, 2.318181818181817455 ) ) ;
#11300=CARTESIAN_POINT ( 'NONE',  ( 10.31249999590322552, 0.5958122406255991210, 5.668774803599163192 ) ) ;
#11309=CARTESIAN_POINT ( 'NONE',  ( 7.000000000000005329, 3.814044456245473835, 4.235925505221166176 ) ) ;
#11316=CARTESIAN_POINT ( 'NONE',  ( 7.843749997951614539, -1.510506337161893864, 4.648860486681943627 ) ) ;
#11325=CARTESIAN_POINT ( 'NONE',  ( 13.00000000000000000, 5.567819778318904511, 1.220402768007685657 ) ) ;
#11333=CARTESIAN_POINT ( 'NONE',  ( 11.46874999795161543, -4.888101187500000222, -3.383411828340740850E-14 ) ) ;
#11337=CARTESIAN_POINT ( 'NONE',  ( -2.000000000000001776, 6.500000000000000000, 0.000000000000000000 ) ) ;
#11358=CIRCLE ( 'NONE', #5589, 5.700000000000001954 ) ;
#11365=CARTESIAN_POINT ( 'NONE',  ( 12.31249999590322552, -5.700000000000001066, -3.945386292505473391E-14 ) ) ;
#11366=CARTESIAN_POINT ( 'NONE',  ( 11.96874999795161365, -3.114526743279282250, 3.846120219227923798 ) ) ;
#11368=EDGE_CURVE ( 'NONE', #17179, #9124, #19681, .T. ) ;
#11373=CARTESIAN_POINT ( 'NONE',  ( 9.000000000000005329, -4.611396867937225252, 3.350375938067065462 ) ) ;
#11382=AXIS2_PLACEMENT_3D ( 'NONE', #8824, #2706, #5803 ) ;
#11386=CARTESIAN_POINT ( 'NONE',  ( 8.968749997951611874, -1.280903732194386579, -4.780397808154273953 ) ) ;
#11387=CARTESIAN_POINT ( 'NONE',  ( 13.00000000000000178, -3.789407127742538517, 3.087705756618167374 ) ) ;
#11390=CARTESIAN_POINT ( 'NONE',  ( 12.50000000000000533, 5.142044285764751699, 2.620002426024544029 ) ) ;
#11403=CARTESIAN_POINT ( 'NONE',  ( 14.84374999795161543, 1.988169868018623720, -4.465502636338010589 ) ) ;
#11410=CARTESIAN_POINT ( 'NONE',  ( 12.31249999590322552, -5.700000000000001066, -3.945386292505473391E-14 ) ) ;
#11427=CARTESIAN_POINT ( 'NONE',  ( 12.96874999795161543, -4.409619785863891472, -2.246813503491864150 ) ) ;
#11466=ORIENTED_EDGE ( 'NONE', *, *, #14853, .F. ) ;
#11480=ORIENTED_EDGE ( 'NONE', *, *, #4568, .T. ) ;
#11482=B_SPLINE_CURVE_WITH_KNOTS ( 'NONE', 3,
 ( #8546, #754, #19050, #14458 ),
 .UNSPECIFIED., .F., .F.,
 ( 4, 4 ),
 ( 0.000000000000000000, 0.001126652051248518789 ),
 .UNSPECIFIED. ) ;
#11500=CARTESIAN_POINT ( 'NONE',  ( 11.34374999795161543, -3.114526743279228072, -3.846120219227966430 ) ) ;
#11506=FACE_OUTER_BOUND ( 'NONE', #6168, .T. ) ;
#11512=DIRECTION ( 'NONE',  ( 0.000000000000000000, -1.224646799147353207E-16, 1.000000000000000000 ) ) ;
#11582=AXIS2_PLACEMENT_3D ( 'NONE', #16493, #73, #16690 ) ;
#11585=CARTESIAN_POINT ( 'NONE',  ( 12.34374999795161543, -1.773574444220693325, -4.620319390059842490 ) ) ;
#11603=CARTESIAN_POINT ( 'NONE',  ( 6.000000000000005329, 4.936344801571289409, 2.850000000000024070 ) ) ;
#11608=CARTESIAN_POINT ( 'NONE',  ( 7.312499995903225525, 0.000000000000000000, -5.700000000000001066 ) ) ;
#11639=DIRECTION ( 'NONE',  ( -1.000000000000000000, -0.000000000000000000, -0.000000000000000000 ) ) ;
#11644=VERTEX_POINT ( 'NONE', #9383 ) ;
#11646=CARTESIAN_POINT ( 'NONE',  ( 8.812499995903225525, -2.620002426024580000, 5.142044285764733935 ) ) ;
#11651=CARTESIAN_POINT ( 'NONE',  ( 6.843749997951615427, 0.000000000000000000, -4.888101187500000222 ) ) ;
#11664=VERTEX_POINT ( 'NONE', #16341 ) ;
#11667=CARTESIAN_POINT ( 'NONE',  ( 7.468749997951615427, 3.270778111535313837, 3.632567103900546712 ) ) ;
#11673=VERTEX_POINT ( 'NONE', #12678 ) ;
#11675=CARTESIAN_POINT ( 'NONE',  ( 13.00000000000000533, -4.057257337410487885, 2.726922038711669494 ) ) ;
#11709=CARTESIAN_POINT ( 'NONE',  ( 12.50000000000000533, -5.142044285764733935, -2.620002426024580000 ) ) ;
#11729=EDGE_CURVE ( 'NONE', #10630, #12192, #18675, .T. ) ;
#11733=PLANE ( 'NONE',  #19362 ) ;
#11734=CARTESIAN_POINT ( 'NONE',  ( 8.968749997951613651, 3.499494075959816541, -3.499494075959816541 ) ) ;
#11740=CARTESIAN_POINT ( 'NONE',  ( 8.968749997951611874, 1.280903732194421218, 4.780397808154266848 ) ) ;
#11746=CARTESIAN_POINT ( 'NONE',  ( 9.500000000000003553, -4.840010801796461593, -3.143139765844656708 ) ) ;
#11756=DIRECTION ( 'NONE',  ( 0.000000000000000000, 0.5000000000000039968, -0.8660254037844363761 ) ) ;
#11764=ORIENTED_EDGE ( 'NONE', *, *, #16940, .T. ) ;
#11766=ADVANCED_FACE ( 'NONE', ( #9034 ), #13008, .T. ) ;
#11775=CARTESIAN_POINT ( 'NONE',  ( 13.00000000000000888, -4.471046188018891421, -1.976722499206046146 ) ) ;
#11776=ORIENTED_EDGE ( 'NONE', *, *, #17717, .F. ) ;
#11778=( BOUNDED_SURFACE ( )  B_SPLINE_SURFACE ( 1, 2, ( 
 ( #400, #14102, #4802, #17207, #17014, #3302, #12706, #11104, #9415, #3499, #6479, #12613, #16825, #13910, #15610, #18603, #509 ),
 ( #9609, #6577, #18801, #10714, #15513, #9216, #1800, #3101, #7893, #105, #14009, #18410, #6379, #4704, #10811, #7798, #12510 ) ),
 .UNSPECIFIED., .F., .F., .F. ) 
 B_SPLINE_SURFACE_WITH_KNOTS ( ( 2, 2 ),
 ( 3, 2, 2, 2, 2, 2, 2, 2, 3 ),
 ( 0.000000000000000000, 1.000000000000000000 ),
 ( 0.000000000000000000, 0.05000000000000000278, 0.1000000000000000056, 0.1499999999999999944, 0.2000000000000000111, 0.2500000000000000000, 0.2999999999999999889, 0.3499999999999999778, 0.4000000000000000222 ),
 .UNSPECIFIED. ) 
 GEOMETRIC_REPRESENTATION_ITEM ( )  RATIONAL_B_SPLINE_SURFACE ( (
 ( 1.000000000000000000, 0.9876883405951377704, 1.000000000000000000, 0.9876883405951377704, 1.000000000000000000, 0.9876883405951377704, 1.000000000000000000, 0.9876883405951377704, 1.000000000000000000, 0.9876883405951377704, 1.000000000000000000, 0.9876883405951377704, 1.000000000000000000, 0.9876883405951377704, 1.000000000000000000, 0.9876883405951377704, 1.000000000000000000),
 ( 1.000000000000000000, 0.9876883405951377704, 1.000000000000000000, 0.9876883405951377704, 1.000000000000000000, 0.9876883405951377704, 1.000000000000000000, 0.9876883405951377704, 1.000000000000000000, 0.9876883405951377704, 1.000000000000000000, 0.9876883405951377704, 1.000000000000000000, 0.9876883405951377704, 1.000000000000000000, 0.9876883405951377704, 1.000000000000000000) ) ) 
 REPRESENTATION_ITEM ( '' )  SURFACE ( )  );
#11800=CARTESIAN_POINT ( 'NONE',  ( 6.843749997951615427, 4.233219804643871598, 2.444050593750020095 ) ) ;
#11801=DIRECTION ( 'NONE',  ( -0.4999999999999978351, -0.7499999999999990008, -0.4330127018922234616 ) ) ;
#11807=CARTESIAN_POINT ( 'NONE',  ( 9.968749997951617203, 4.409619785863906571, -2.246813503491833508 ) ) ;
#11815=CARTESIAN_POINT ( 'NONE',  ( 6.968749997951614539, 0.7741991708318887166, -4.888101187500000222 ) ) ;
#11830=CARTESIAN_POINT ( 'NONE',  ( 10.81249999590322375, 4.840010801796481132, 3.143139765844622957 ) ) ;
#11865=CARTESIAN_POINT ( 'NONE',  ( 9.468749997951615427, 0.5109457054261445919, 4.861323657744411442 ) ) ;
#11866=VERTEX_POINT ( 'NONE', #2821 ) ;
#11883=ORIENTED_EDGE ( 'NONE', *, *, #703, .T. ) ;
#11890=AXIS2_PLACEMENT_3D ( 'NONE', #13126, #3525, #6708 ) ;
#11899=CARTESIAN_POINT ( 'NONE',  ( 10.81249999590322375, -0.3020334839682879413, 5.763142191869155440 ) ) ;
#11917=CARTESIAN_POINT ( 'NONE',  ( 10.34374999795161543, 4.409619785863906571, -2.246813503491833508 ) ) ;
#11930=CARTESIAN_POINT ( 'NONE',  ( 8.843749997951615427, 4.861323657744407001, 0.5109457054261780096 ) ) ;
#11935=ORIENTED_EDGE ( 'NONE', *, *, #5520, .F. ) ;
#11939=CIRCLE ( 'NONE', #1402, 4.400000000000000355 ) ;
#11942=CARTESIAN_POINT ( 'NONE',  ( 12.46874999795161543, -1.016293382781378485, -4.781284448697201483 ) ) ;
#11943=CARTESIAN_POINT ( 'NONE',  ( 13.00000000000000178, 0.5236311934647676081, 4.860400829920955346 ) ) ;
#11953=CARTESIAN_POINT ( 'NONE',  ( 10.00000000000000533, 5.421022142882375938, -1.761396867937200739 ) ) ;
#11979=CARTESIAN_POINT ( 'NONE',  ( 13.31249999590322730, 5.421022142882376826, 1.761396867937200073 ) ) ;
#11998=CARTESIAN_POINT ( 'NONE',  ( 10.64522241986047568, 2.725425358843983450E-16, 5.700000000000002842 ) ) ;
#12001=CARTESIAN_POINT ( 'NONE',  ( 9.812499995903223748, -5.574407415329147852, -1.493657965219562511 ) ) ;
#12018=( BOUNDED_CURVE ( )  B_SPLINE_CURVE ( 2, ( #5528, #17739, #10144, #7111, #13242, #11734, #4722, #5915, #7714, #1620, #18044, #1324, #16540, #12233, #1528 ),
 .UNSPECIFIED., .F., .F. ) 
 B_SPLINE_CURVE_WITH_KNOTS ( ( 3, 2, 2, 2, 2, 2, 2, 3 ),
 ( 0.000000000000000000, 0.05000000000000000971, 0.1000000000000000194, 0.1499999999999999944, 0.2000000000000000389, 0.2500000000000000000, 0.2999999999999999889, 0.3265529187307102399 ),
 .UNSPECIFIED. ) 
 CURVE ( )  GEOMETRIC_REPRESENTATION_ITEM ( )  RATIONAL_B_SPLINE_CURVE ( ( 1.000000000000000000, 0.9876883405951377704, 1.000000000000000000, 0.9876883405951377704, 1.000000000000000000, 0.9876883405951377704, 1.000000000000000000, 0.9876883405951377704, 1.000000000000000000, 0.9876883405951377704, 1.000000000000000000, 0.9876883405951377704, 1.000000000000000000, 0.9934617901676501273, 0.9938679225082089896 ) ) 
 REPRESENTATION_ITEM ( '' )  );
#12031=ORIENTED_EDGE ( 'NONE', *, *, #4043, .F. ) ;
#12046=CARTESIAN_POINT ( 'NONE',  ( 9.000000000000005329, -5.207209108562803834, -2.318398865532109721 ) ) ;
#12047=CARTESIAN_POINT ( 'NONE',  ( 13.00000000000000178, 0.5876048313370836329, 4.852654302691283839 ) ) ;
#12052=CARTESIAN_POINT ( 'NONE',  ( 13.00000000000000178, 0.000000000000000000, 0.000000000000000000 ) ) ;
#12055=CARTESIAN_POINT ( 'NONE',  ( 13.00000000000000178, 3.789407127742559833, -3.087705756618140285 ) ) ;
#12057=ORIENTED_EDGE ( 'NONE', *, *, #14193, .T. ) ;
#12062=CARTESIAN_POINT ( 'NONE',  ( 12.46874999795161543, -1.016293382781378485, -4.781284448697201483 ) ) ;
#12068=CARTESIAN_POINT ( 'NONE',  ( 2.999999999999998224, 0.000000000000000000, 0.000000000000000000 ) ) ;
#12073=ORIENTED_EDGE ( 'NONE', *, *, #11368, .T. ) ;
#12079=VECTOR ( 'NONE', #19584, 1000.000000000000000 ) ;
#12082=EDGE_CURVE ( 'NONE', #9272, #5021, #10222, .T. ) ;
#12091=CIRCLE ( 'NONE', #2820, 5.700000000000001954 ) ;
#12102=CARTESIAN_POINT ( 'NONE',  ( 6.968749997951614539, -3.846120219227901149, -3.114526743279308896 ) ) ;
#12108=ORIENTED_EDGE ( 'NONE', *, *, #1468, .F. ) ;
#12112=CARTESIAN_POINT ( 'NONE',  ( 12.00000000000000533, -5.421022142882365280, -1.761396867937238042 ) ) ;
#12115=DIRECTION ( 'NONE',  ( 0.000000000000000000, -0.6818181818181822118, 0.7315216790650489465 ) ) ;
#12124=EDGE_CURVE ( 'NONE', #7035, #8351, #6298, .T. ) ;
#12134=CARTESIAN_POINT ( 'NONE',  ( 9.843749997951615427, 4.465502636338024800, 1.988169868018593300 ) ) ;
#12141=AXIS2_PLACEMENT_3D ( 'NONE', #2046, #8151, #10859 ) ;
#12161=CARTESIAN_POINT ( 'NONE',  ( 13.00000000000000000, -0.2080849974988778772, -4.883670121236158401 ) ) ;
#12170=CARTESIAN_POINT ( 'NONE',  ( 10.84374999795161543, 4.648860486681953397, -1.510506337161861667 ) ) ;
#12177=CARTESIAN_POINT ( 'NONE',  ( 11.81249999590322552, 5.699999999999999289, -0.9027913098498572264 ) ) ;
#12190=AXIS2_PLACEMENT_3D ( 'NONE', #14239, #8020, #9244 ) ;
#12192=VERTEX_POINT ( 'NONE', #8319 ) ;
#12197=CARTESIAN_POINT ( 'NONE',  ( 6.000000000000005329, -4.936344801571327601, 2.849999999999954348 ) ) ;
#12204=AXIS2_PLACEMENT_3D ( 'NONE', #6361, #7781, #9395 ) ;
#12220=EDGE_CURVE ( 'NONE', #19560, #4381, #5001, .T. ) ;
#12222=CARTESIAN_POINT ( 'NONE',  ( 8.843749997951615427, -2.873153789725853002, 3.954556930911842016 ) ) ;
#12232=CARTESIAN_POINT ( 'NONE',  ( 7.843749997951614539, 4.781284448697194378, -1.016293382781411569 ) ) ;
#12233=CARTESIAN_POINT ( 'NONE',  ( 12.73273607671833929, 4.522548057701235358, 1.899256020376435927 ) ) ;
#12282=ORIENTED_EDGE ( 'NONE', *, *, #16350, .F. ) ;
#12285=SURFACE_SIDE_STYLE ('',( #19580 ) ) ;
#12290=CARTESIAN_POINT ( 'NONE',  ( 13.00000000000000000, -5.567819778318897406, -1.220402768007724292 ) ) ;
#12304=CARTESIAN_POINT ( 'NONE',  ( 9.968749997951615427, 0.2590123213421660631, -4.942249507334554259 ) ) ;
#12326=DIRECTION ( 'NONE',  ( -1.000000000000000000, 0.000000000000000000, 0.000000000000000000 ) ) ;
#12345=CARTESIAN_POINT ( 'NONE',  ( 8.968749997951613651, 4.780397808154257078, 1.280903732194454303 ) ) ;
#12356=ORIENTED_EDGE ( 'NONE', *, *, #12124, .T. ) ;
#12358=CARTESIAN_POINT ( 'NONE',  ( 13.34374999795161365, 4.150607464521828938, -2.695436003842674566 ) ) ;
#12374=ORIENTED_EDGE ( 'NONE', *, *, #9084, .F. ) ;
#12376=EDGE_CURVE ( 'NONE', #7834, #4794, #9412, .T. ) ;
#12378=CARTESIAN_POINT ( 'NONE',  ( 8.843749997951615427, 1.988169868018562436, 4.465502636338039011 ) ) ;
#12386=ORIENTED_EDGE ( 'NONE', *, *, #7445, .F. ) ;
#12396=CARTESIAN_POINT ( 'NONE',  ( 8.843749997951615427, -1.988169868018530462, -4.465502636338051445 ) ) ;
#12404=CARTESIAN_POINT ( 'NONE',  ( -2.000000000000001776, -3.218695387886215009, -3.000000000000002220 ) ) ;
#12413=PLANE ( 'NONE',  #10338 ) ;
#12416=ORIENTED_EDGE ( 'NONE', *, *, #14058, .T. ) ;
#12425=CARTESIAN_POINT ( 'NONE',  ( 8.812499995903225525, 2.620002426024544029, -5.142044285764751699 ) ) ;
#12426=( BOUNDED_CURVE ( )  B_SPLINE_CURVE ( 2, ( #10916, #17020, #3309, #17119, #9423, #308, #6389, #13719, #18611, #12910, #2006, #611, #2297, #8507, #8104 ),
 .UNSPECIFIED., .F., .F. ) 
 B_SPLINE_CURVE_WITH_KNOTS ( ( 3, 2, 2, 2, 2, 2, 2, 3 ),
 ( 0.000000000000000000, 0.04999999999999999584, 0.09999999999999999167, 0.1499999999999999944, 0.1999999999999999833, 0.2500000000000000000, 0.2999999999999999889, 0.3499999999999999778 ),
 .UNSPECIFIED. ) 
 CURVE ( )  GEOMETRIC_REPRESENTATION_ITEM ( )  RATIONAL_B_SPLINE_CURVE ( ( 1.000000000000000000, 0.9876883405951377704, 1.000000000000000000, 0.9876883405951377704, 1.000000000000000000, 0.9876883405951377704, 1.000000000000000000, 0.9876883405951377704, 1.000000000000000000, 0.9876883405951377704, 1.000000000000000000, 0.9876883405951377704, 1.000000000000000000, 0.9876883405951377704, 1.000000000000000000 ) ) 
 REPRESENTATION_ITEM ( '' )  );
#12432=ORIENTED_EDGE ( 'NONE', *, *, #14032, .T. ) ;
#12440=PRODUCT_DEFINITION_FORMATION_WITH_SPECIFIED_SOURCE ( 'ANY', '', #5221, .NOT_KNOWN. ) ;
#12452=CARTESIAN_POINT ( 'NONE',  ( 12.84374999795161543, 3.632567103900569361, -3.270778111535288080 ) ) ;
#12458=DIRECTION ( 'NONE',  ( 0.000000000000000000, 0.000000000000000000, 1.000000000000000000 ) ) ;
#12472=DIRECTION ( 'NONE',  ( -1.000000000000000000, 0.000000000000000000, -0.000000000000000000 ) ) ;
#12480=ORIENTED_EDGE ( 'NONE', *, *, #5716, .F. ) ;
#12491=CARTESIAN_POINT ( 'NONE',  ( 6.843749997951615427, -3.413342815706642518E-14, 4.888101187500000222 ) ) ;
#12492=VECTOR ( 'NONE', #1549, 1000.000000000000000 ) ;
#12495=CARTESIAN_POINT ( 'NONE',  ( 14.84374999795161543, 1.988169868018623720, -4.465502636338010589 ) ) ;
#12498=EDGE_CURVE ( 'NONE', #6403, #12192, #10904, .T. ) ;
#12501=LINE ( 'NONE', #4600, #12991 ) ;
#12508=AXIS2_PLACEMENT_3D ( 'NONE', #14730, #11234, #2417 ) ;
#12510=CARTESIAN_POINT ( 'NONE',  ( 14.00000000000000533, -2.318398865532073305, 5.207209108562820710 ) ) ;
#12518=CARTESIAN_POINT ( 'NONE',  ( 13.84374999795161543, -3.954556930911842016, -2.873153789725852558 ) ) ;
#12526=CARTESIAN_POINT ( 'NONE',  ( 13.00000000000000178, 4.920309236097874184, 1.604440756441510407 ) ) ;
#12527=ORIENTED_EDGE ( 'NONE', *, *, #13159, .T. ) ;
#12545=DIRECTION ( 'NONE',  ( 1.000000000000000000, -0.000000000000000000, -0.000000000000000000 ) ) ;
#12558=CIRCLE ( 'NONE', #14101, 4.400000000000000355 ) ;
#12559=ORIENTED_EDGE ( 'NONE', *, *, #4418, .F. ) ;
#12574=ORIENTED_EDGE ( 'NONE', *, *, #1468, .T. ) ;
#12583=ORIENTED_EDGE ( 'NONE', *, *, #2688, .T. ) ;
#12592=( GEOMETRIC_REPRESENTATION_CONTEXT ( 3 ) GLOBAL_UNCERTAINTY_ASSIGNED_CONTEXT ( ( #802 ) ) GLOBAL_UNIT_ASSIGNED_CONTEXT ( ( #13780, #8982, #16888 ) ) REPRESENTATION_CONTEXT ( 'NONE', 'WORKASPACE' ) );
#12599=CARTESIAN_POINT ( 'NONE',  ( 8.843749997951615427, -4.861323657744403448, -0.5109457054262123155 ) ) ;
#12601=CARTESIAN_POINT ( 'NONE',  ( 13.00000000000000000, 4.125339889944109828, -2.622041954598519187 ) ) ;
#12610=CARTESIAN_POINT ( 'NONE',  ( 7.812499995903224637, 5.387740456496234565, -2.068159791354183596 ) ) ;
#12613=CARTESIAN_POINT ( 'NONE',  ( 11.96874999795161365, 1.773574444220725299, 4.620319390059829168 ) ) ;
#12617=CYLINDRICAL_SURFACE ( 'NONE', #897, 5.700000000000001954 ) ;
#12618=ORIENTED_EDGE ( 'NONE', *, *, #13365, .F. ) ;
#12619=CARTESIAN_POINT ( 'NONE',  ( 14.34374999795161365, -3.499494075959791672, -3.499494075959840078 ) ) ;
#12622=PRODUCT_DEFINITION ( 'UNKNOWN', '', #12440, #1388 ) ;
#12624=CARTESIAN_POINT ( 'NONE',  ( 13.00000000000000178, 3.789407127742559833, -3.087705756618140285 ) ) ;
#12625=CARTESIAN_POINT ( 'NONE',  ( 9.812499995903225525, 4.080749450109650844, -4.080749450109650844 ) ) ;
#12635=EDGE_LOOP ( 'NONE', ( #8064, #6797, #12282, #12527 ) ) ;
#12651=ORIENTED_EDGE ( 'NONE', *, *, #18251, .F. ) ;
#12653=CARTESIAN_POINT ( 'NONE',  ( 8.000000000000005329, -5.668774803599153422, -0.5958122406256771697 ) ) ;
#12654=CARTESIAN_POINT ( 'NONE',  ( 11.31249999590322375, 1.185096637661293251, -5.575441324182679459 ) ) ;
#12658=ORIENTED_EDGE ( 'NONE', *, *, #914, .T. ) ;
#12661=CARTESIAN_POINT ( 'NONE',  ( 9.343749997951615427, 4.780397808154257078, 1.280903732194454303 ) ) ;
#12678=CARTESIAN_POINT ( 'NONE',  ( 13.00000000000000000, -0.2080849974988778772, -4.883670121236158401 ) ) ;
#12684=CARTESIAN_POINT ( 'NONE',  ( 13.00000000000000000, 4.125339889944109828, -2.622041954598519187 ) ) ;
#12687=CARTESIAN_POINT ( 'NONE',  ( 10.84374999795161543, 1.016293382781477961, -4.781284448697179279 ) ) ;
#12697=CARTESIAN_POINT ( 'NONE',  ( 8.343749997951613651, 4.942249507334556924, -0.2590123213420975623 ) ) ;
#12706=CARTESIAN_POINT ( 'NONE',  ( 9.468749997951615427, 4.465502636338023912, 1.988169868018593300 ) ) ;
#12714=CARTESIAN_POINT ( 'NONE',  ( 8.312499995903225525, -1.761396867937238486, 5.421022142882364392 ) ) ;
#12718=EDGE_CURVE ( 'NONE', #1853, #2859, #4089, .T. ) ;
#12728=CARTESIAN_POINT ( 'NONE',  ( 7.968749997951616315, -2.246813503491864150, 4.409619785863891472 ) ) ;
#12751=CARTESIAN_POINT ( 'NONE',  ( 9.843749997951615427, 0.5109457054261445919, 4.861323657744411442 ) ) ;
#12756=CARTESIAN_POINT ( 'NONE',  ( 9.843749997951615427, 0.5109457054261445919, 4.861323657744411442 ) ) ;
#12758=CARTESIAN_POINT ( 'NONE',  ( 11.34374999795161543, 3.114526743279255161, 3.846120219227944670 ) ) ;
#12763=CARTESIAN_POINT ( 'NONE',  ( 7.468749997951615427, 3.270778111535313837, 3.632567103900546712 ) ) ;
#12766=AXIS2_PLACEMENT_3D ( 'NONE', #19255, #11756, #18966 ) ;
#12770=CARTESIAN_POINT ( 'NONE',  ( 11.50000000000000355, 2.068159791354183596, 5.387740456496233676 ) ) ;
#12774=PLANE ( 'NONE',  #139 ) ;
#12778=CARTESIAN_POINT ( 'NONE',  ( -2.000000000000001776, 0.000000000000000000, 0.000000000000000000 ) ) ;
#12783=CARTESIAN_POINT ( 'NONE',  ( 13.00000000000000000, 4.091807895435353615, -2.674798881044243792 ) ) ;
#12787=CARTESIAN_POINT ( 'NONE',  ( 12.34374999795161543, -4.888101187499994893, -0.7741991708319226895 ) ) ;
#12791=CARTESIAN_POINT ( 'NONE',  ( 6.000000000000005329, 0.000000000000000000, -5.700000000000001066 ) ) ;
#12804=CARTESIAN_POINT ( 'NONE',  ( 13.96874999795161365, -4.780397808154265960, 1.280903732194421663 ) ) ;
#12825=FACE_OUTER_BOUND ( 'NONE', #14511, .T. ) ;
#12828=VERTEX_POINT ( 'NONE', #12290 ) ;
#12847=FACE_BOUND ( 'NONE', #1595, .T. ) ;
#12848=CARTESIAN_POINT ( 'NONE',  ( 13.00000000000000178, -0.3952618871915391519, -4.872094134945741395 ) ) ;
#12855=CARTESIAN_POINT ( 'NONE',  ( 8.343749997951611874, 2.695436003842704764, 4.150607464521812062 ) ) ;
#12856=CARTESIAN_POINT ( 'NONE',  ( 11.96874999795161365, 1.773574444220725299, 4.620319390059829168 ) ) ;
#12861=CARTESIAN_POINT ( 'NONE',  ( 10.96874999795161720, -1.773574444220757496, 4.620319390059819398 ) ) ;
#12868=CARTESIAN_POINT ( 'NONE',  ( 13.00000000000000533, -0.5958122406256377568, 5.668774803599156975 ) ) ;
#12870=CARTESIAN_POINT ( 'NONE',  ( 10.50000000000000533, -5.700000000000006395, 0.9027913098498173694 ) ) ;
#12875=SURFACE_SIDE_STYLE ('',( #17768 ) ) ;
#12884=ORIENTED_EDGE ( 'NONE', *, *, #18367, .F. ) ;
#12886=CARTESIAN_POINT ( 'NONE',  ( 9.468749997951615427, -0.5109457054261099529, -4.861323657744413218 ) ) ;
#12887=CARTESIAN_POINT ( 'NONE',  ( 12.84374999795161543, 3.632567103900569361, -3.270778111535288080 ) ) ;
#12890=CARTESIAN_POINT ( 'NONE',  ( 8.000000000000005329, 3.350375938067097437, -4.611396867937201272 ) ) ;
#12906=CARTESIAN_POINT ( 'NONE',  ( 10.84374999795161543, -3.632567103900500971, -3.270778111535363131 ) ) ;
#12909=ORIENTED_EDGE ( 'NONE', *, *, #5716, .T. ) ;
#12910=CARTESIAN_POINT ( 'NONE',  ( 10.50000000000000533, 2.068159791354258648, -5.387740456496205255 ) ) ;
#12925=CARTESIAN_POINT ( 'NONE',  ( 8.968749997951611874, -3.499494075959840966, 3.499494075959791672 ) ) ;
#12941=CIRCLE ( 'NONE', #7163, 4.400000000000000355 ) ;
#12960=( BOUNDED_CURVE ( )  B_SPLINE_CURVE ( 2, ( #8563, #9979, #14672, #10464, #4258, #10562, #4453, #3045, #16568, #19453, #16660, #17968, #12062, #1253, #12161 ),
 .UNSPECIFIED., .F., .F. ) 
 B_SPLINE_CURVE_WITH_KNOTS ( ( 3, 2, 2, 2, 2, 2, 2, 3 ),
 ( 0.000000000000000000, 0.05000000000000000971, 0.1000000000000000194, 0.1499999999999999944, 0.2000000000000000389, 0.2500000000000000000, 0.2999999999999999889, 0.3265529187307102399 ),
 .UNSPECIFIED. ) 
 CURVE ( )  GEOMETRIC_REPRESENTATION_ITEM ( )  RATIONAL_B_SPLINE_CURVE ( ( 1.000000000000000000, 0.9876883405951377704, 1.000000000000000000, 0.9876883405951377704, 1.000000000000000000, 0.9876883405951377704, 1.000000000000000000, 0.9876883405951377704, 1.000000000000000000, 0.9876883405951377704, 1.000000000000000000, 0.9876883405951377704, 1.000000000000000000, 0.9934617901676501273, 0.9938679225082089896 ) ) 
 REPRESENTATION_ITEM ( '' )  );
#12986=CARTESIAN_POINT ( 'NONE',  ( 6.468749997951615427, -4.233219804643852946, -2.444050593750049849 ) ) ;
#12987=CARTESIAN_POINT ( 'NONE',  ( 13.00000000000000000, -4.125339889944092953, 2.622041954598548941 ) ) ;
#12991=VECTOR ( 'NONE', #18597, 1000.000000000000114 ) ;
#12995=CARTESIAN_POINT ( 'NONE',  ( 12.84374999795161543, 1.016293382781411792, 4.781284448697195266 ) ) ;
#13006=CARTESIAN_POINT ( 'NONE',  ( 9.468749997951615427, -4.465502636338009701, -1.988169868018624609 ) ) ;
#13008=TOROIDAL_SURFACE ( 'NONE', #13322, -32.79058411375427795, 40.00000000000000711 ) ;
#13015=DIRECTION ( 'NONE',  ( 0.000000000000000000, -1.000000000000000000, 0.000000000000000000 ) ) ;
#13028=CARTESIAN_POINT ( 'NONE',  ( 8.812499995903225525, -5.763142191869158992, 0.3020334839682081163 ) ) ;
#13040=LINE ( 'NONE', #5521, #1334 ) ;
#13052=VECTOR ( 'NONE', #17897, 1000.000000000000000 ) ;
#13058=DIRECTION ( 'NONE',  ( 0.000000000000000000, 0.6818181818181816567, -0.7315216790650493905 ) ) ;
#13065=CARTESIAN_POINT ( 'NONE',  ( 12.99999999999998757, -0.02830770314431023046, 5.175540411820490405 ) ) ;
#13069=( BOUNDED_SURFACE ( )  B_SPLINE_SURFACE ( 1, 2, ( 
 ( #15211, #16313, #7181, #10414, #19404, #5691, #16513, #11807, #8905, #15009, #1300, #7379, #7791, #7587, #9408, #10802, #6281 ),
 ( #10707, #16912, #4698, #4990, #7687, #1596, #15407, #6374, #11097, #3191, #16818, #14092, #3092, #17200, #13904, #9603, #6184 ) ),
 .UNSPECIFIED., .F., .F., .F. ) 
 B_SPLINE_SURFACE_WITH_KNOTS ( ( 2, 2 ),
 ( 3, 2, 2, 2, 2, 2, 2, 2, 3 ),
 ( 0.000000000000000000, 1.000000000000000000 ),
 ( 0.000000000000000000, 0.05000000000000000278, 0.1000000000000000056, 0.1499999999999999944, 0.2000000000000000111, 0.2500000000000000000, 0.2999999999999999889, 0.3499999999999999778, 0.4000000000000000222 ),
 .UNSPECIFIED. ) 
 GEOMETRIC_REPRESENTATION_ITEM ( )  RATIONAL_B_SPLINE_SURFACE ( (
 ( 1.000000000000000000, 0.9876883405951377704, 1.000000000000000000, 0.9876883405951377704, 1.000000000000000000, 0.9876883405951377704, 1.000000000000000000, 0.9876883405951377704, 1.000000000000000000, 0.9876883405951377704, 1.000000000000000000, 0.9876883405951377704, 1.000000000000000000, 0.9876883405951377704, 1.000000000000000000, 0.9876883405951377704, 1.000000000000000000),
 ( 1.000000000000000000, 0.9876883405951377704, 1.000000000000000000, 0.9876883405951377704, 1.000000000000000000, 0.9876883405951377704, 1.000000000000000000, 0.9876883405951377704, 1.000000000000000000, 0.9876883405951377704, 1.000000000000000000, 0.9876883405951377704, 1.000000000000000000, 0.9876883405951377704, 1.000000000000000000, 0.9876883405951377704, 1.000000000000000000) ) ) 
 REPRESENTATION_ITEM ( '' )  SURFACE ( )  );
#13081=CARTESIAN_POINT ( 'NONE',  ( 11.84374999795161365, 2.444050593750049405, -4.233219804643852946 ) ) ;
#13105=ORIENTED_EDGE ( 'NONE', *, *, #6311, .T. ) ;
#13126=CARTESIAN_POINT ( 'NONE',  ( 2.999999999999998224, 2.487173708821167839, -2.318181818181817899 ) ) ;
#13143=ORIENTED_EDGE ( 'NONE', *, *, #11189, .F. ) ;
#13147=ORIENTED_EDGE ( 'NONE', *, *, #18623, .F. ) ;
#13159=EDGE_CURVE ( 'NONE', #9124, #9454, #12091, .T. ) ;
#13175=CARTESIAN_POINT ( 'NONE',  ( 12.96874999795161543, -4.150607464521812062, 2.695436003842704764 ) ) ;
#13190=CARTESIAN_POINT ( 'NONE',  ( 13.00000000000000178, 0.7793280607715257213, 4.825575716215943167 ) ) ;
#13209=DIRECTION ( 'NONE',  ( 0.000000000000000000, 0.000000000000000000, 1.000000000000000000 ) ) ;
#13226=PRODUCT_DEFINITION_SHAPE ( 'NONE', 'NONE',  #12622 ) ;
#13227=LINE ( 'NONE', #17924, #16682 ) ;
#13230=VECTOR ( 'NONE', #16883, 1000.000000000000000 ) ;
#13232=CARTESIAN_POINT ( 'NONE',  ( 10.64522241986047568, 2.725425358843983450E-16, 5.700000000000002842 ) ) ;
#13242=CARTESIAN_POINT ( 'NONE',  ( 8.468749997951615427, 2.873153789725825469, -3.954556930911862000 ) ) ;
#13256=FACE_OUTER_BOUND ( 'NONE', #13555, .T. ) ;
#13261=CARTESIAN_POINT ( 'NONE',  ( 8.500000000000005329, 4.080749450109650844, -4.080749450109650844 ) ) ;
#13277=CARTESIAN_POINT ( 'NONE',  ( 13.00000000000000000, -4.091807895435336739, 2.674798881044273546 ) ) ;
#13286=ORIENTED_EDGE ( 'NONE', *, *, #15075, .T. ) ;
#13297=CARTESIAN_POINT ( 'NONE',  ( 9.343749997951615427, 1.280903732194421218, 4.780397808154266848 ) ) ;
#13306=CARTESIAN_POINT ( 'NONE',  ( 10.50000000000000711, -5.700000000000005507, 0.9027913098498173694 ) ) ;
#13322=AXIS2_PLACEMENT_3D ( 'NONE', #15137, #9237, #7308 ) ;
#13328=CARTESIAN_POINT ( 'NONE',  ( 11.81249999590322552, 3.631840208645794821, 4.484949146646379781 ) ) ;
#13332=CARTESIAN_POINT ( 'NONE',  ( 2.999999999999998224, 3.950217066951266176, 3.681818181818181213 ) ) ;
#13339=CARTESIAN_POINT ( 'NONE',  ( 8.968749997951611874, -4.780397808154247308, -1.280903732194487166 ) ) ;
#13347=ORIENTED_EDGE ( 'NONE', *, *, #7855, .F. ) ;
#13363=CARTESIAN_POINT ( 'NONE',  ( 10.46874999795161720, -1.016293382781444654, 4.781284448697187273 ) ) ;
#13365=EDGE_CURVE ( 'NONE', #13931, #4794, #9966, .T. ) ;
#13388=FACE_OUTER_BOUND ( 'NONE', #3768, .T. ) ;
#13394=CARTESIAN_POINT ( 'NONE',  ( 13.31249999590322730, -4.235925505221167064, 3.814044456245474279 ) ) ;
#13396=CARTESIAN_POINT ( 'NONE',  ( 12.81249999590322552, -2.068159791354146293, -5.387740456496247887 ) ) ;
#13397=DIRECTION ( 'NONE',  ( 1.000000000000000000, -0.000000000000000000, -0.000000000000000000 ) ) ;
#13408=CARTESIAN_POINT ( 'NONE',  ( 8.468749997951615427, 2.873153789725825469, -3.954556930911862000 ) ) ;
#13423=CARTESIAN_POINT ( 'NONE',  ( 11.34374999795161543, 3.114526743279256493, 3.846120219227944670 ) ) ;
#13435=CARTESIAN_POINT ( 'NONE',  ( 10.50000000000000711, -3.631840208645764179, -4.484949146646406426 ) ) ;
#13458=CARTESIAN_POINT ( 'NONE',  ( 10.50000000000000711, -2.068159791354221344, 5.387740456496221242 ) ) ;
#13472=CARTESIAN_POINT ( 'NONE',  ( 7.312499995903225525, 0.000000000000000000, -5.700000000000001066 ) ) ;
#13480=CARTESIAN_POINT ( 'NONE',  ( 7.078124996927420476, -3.696815770993907903E-14, 5.294050593750000644 ) ) ;
#13495=CARTESIAN_POINT ( 'NONE',  ( 15.31249999590322552, 2.318398865532109276, -5.207209108562804722 ) ) ;
#13504=CARTESIAN_POINT ( 'NONE',  ( 2.999999999999998224, -3.218695387886217674, 2.999999999999999112 ) ) ;
#13505=CIRCLE ( 'NONE', #5503, 4.400000000000000355 ) ;
#13507=VERTEX_POINT ( 'NONE', #10446 ) ;
#13511=CARTESIAN_POINT ( 'NONE',  ( 11.84374999795161365, 4.888101187500000222, -2.993098736590125853E-16 ) ) ;
#13528=CARTESIAN_POINT ( 'NONE',  ( 14.84374999795161543, -1.988169868018592412, 4.465502636338025688 ) ) ;
#13540=CARTESIAN_POINT ( 'NONE',  ( 12.00000000000000533, -1.185096637661177343, -5.575441324182703440 ) ) ;
#13555=EDGE_LOOP ( 'NONE', ( #13892, #16033, #4940, #18584 ) ) ;
#13577=CARTESIAN_POINT ( 'NONE',  ( 8.312499995903225525, 1.761396867937200517, -5.421022142882375938 ) ) ;
#13597=CARTESIAN_POINT ( 'NONE',  ( 14.31249999590322552, -5.207209108562836697, 2.318398865532038666 ) ) ;
#13602=CARTESIAN_POINT ( 'NONE',  ( 8.000000000000005329, 5.668774803599156975, 0.5958122406256382009 ) ) ;
#13606=CARTESIAN_POINT ( 'NONE',  ( 6.000000000000005329, 4.936344801571308061, -2.849999999999988987 ) ) ;
#13610=CARTESIAN_POINT ( 'NONE',  ( 12.31249999590322552, -2.849999999999954792, -4.936344801571327601 ) ) ;
#13611=CARTESIAN_POINT ( 'NONE',  ( 13.96874999795161365, -4.780397808154265960, 1.280903732194421663 ) ) ;
#13613=CARTESIAN_POINT ( 'NONE',  ( 6.468749997951615427, -3.413342815706642518E-14, 4.888101187500000222 ) ) ;
#13614=CARTESIAN_POINT ( 'NONE',  ( 6.843749997951615427, 0.000000000000000000, -4.888101187500000222 ) ) ;
#13640=CARTESIAN_POINT ( 'NONE',  ( 10.46874999795161720, -3.632567103900500971, -3.270778111535363131 ) ) ;
#13643=VERTEX_POINT ( 'NONE', #14207 ) ;
#13668=CARTESIAN_POINT ( 'NONE',  ( 7.343749997951615427, 0.7741991708318887166, -4.888101187500000222 ) ) ;
#13678=CARTESIAN_POINT ( 'NONE',  ( 9.843749997951615427, 3.954556930911862000, -2.873153789725825469 ) ) ;
#13691=CARTESIAN_POINT ( 'NONE',  ( 13.00000000000000178, 4.568735188514060575, 1.737869959597756697 ) ) ;
#13695=ORIENTED_EDGE ( 'NONE', *, *, #2480, .F. ) ;
#13713=CARTESIAN_POINT ( 'NONE',  ( 12.96874999795161543, 4.409619785863906571, 2.246813503491833508 ) ) ;
#13718=ORIENTED_EDGE ( 'NONE', *, *, #1247, .T. ) ;
#13719=CARTESIAN_POINT ( 'NONE',  ( 9.500000000000005329, 0.3020334839683282424, -5.763142191869152775 ) ) ;
#13726=CARTESIAN_POINT ( 'NONE',  ( 7.343749997951615427, 4.620319390059830056, -1.773574444220725521 ) ) ;
#13734=ORIENTED_EDGE ( 'NONE', *, *, #3812, .F. ) ;
#13740=CARTESIAN_POINT ( 'NONE',  ( 10.96874999795161720, 3.114526743279255161, 3.846120219227944670 ) ) ;
#13756=ORIENTED_EDGE ( 'NONE', *, *, #3812, .T. ) ;
#13780=( LENGTH_UNIT ( ) NAMED_UNIT ( * ) SI_UNIT ( .MILLI., .METRE. ) );
#13790=ORIENTED_EDGE ( 'NONE', *, *, #14476, .F. ) ;
#13794=CARTESIAN_POINT ( 'NONE',  ( 8.000000000000005329, -2.318398865532001363, -5.207209108562852684 ) ) ;
#13797=CARTESIAN_POINT ( 'NONE',  ( 7.468749997951615427, -3.270778111535287191, -3.632567103900569361 ) ) ;
#13800=VECTOR ( 'NONE', #15788, 1000.000000000000114 ) ;
#13807=CARTESIAN_POINT ( 'NONE',  ( 14.34374999795161365, -4.780397808154265960, 1.280903732194421663 ) ) ;
#13811=ADVANCED_FACE ( 'NONE', ( #704 ), #9626, .F. ) ;
#13816=CARTESIAN_POINT ( 'NONE',  ( 8.968749997951611874, -3.499494075959840966, 3.499494075959791672 ) ) ;
#13842=CARTESIAN_POINT ( 'NONE',  ( 13.00000000000000000, -1.727010089215899713, -5.432074755721473025 ) ) ;
#13853=CARTESIAN_POINT ( 'NONE',  ( 8.500000000000005329, -5.574407415329147852, -1.493657965219562511 ) ) ;
#13854=CARTESIAN_POINT ( 'NONE',  ( 15.31249999590322552, 5.668774803599165857, -0.5958122406255597081 ) ) ;
#13877=CARTESIAN_POINT ( 'NONE',  ( 7.343749997951615427, 3.846120219227923798, 3.114526743279282694 ) ) ;
#13892=ORIENTED_EDGE ( 'NONE', *, *, #13365, .T. ) ;
#13893=CARTESIAN_POINT ( 'NONE',  ( 7.343749997951615427, -3.846120219227901149, -3.114526743279308896 ) ) ;
#13894=CARTESIAN_POINT ( 'NONE',  ( 13.00000000000000000, -4.362347728716193807, -2.206210144330614131 ) ) ;
#13904=CARTESIAN_POINT ( 'NONE',  ( 13.00000000000000533, 4.611396867937201272, 3.350375938067096548 ) ) ;
#13910=CARTESIAN_POINT ( 'NONE',  ( 12.96874999795161543, 0.2590123213420971182, 4.942249507334556924 ) ) ;
#13918=CARTESIAN_POINT ( 'NONE',  ( 10.34374999795161543, -4.409619785863921670, 2.246813503491803310 ) ) ;
#13931=VERTEX_POINT ( 'NONE', #5058 ) ;
#13946=AXIS2_PLACEMENT_3D ( 'NONE', #6788, #13015, #2485 ) ;
#13950=EDGE_LOOP ( 'NONE', ( #19076, #17029, #10133, #2143, #10286, #5245, #9925, #13756, #6303, #12432, #19670, #1501, #10082, #17941, #5978, #4208, #1517, #4372, #17365, #17441, #17158, #13286, #12574, #1718 ) ) ;
#13952=CARTESIAN_POINT ( 'NONE',  ( 13.81249999590322552, 4.840010801796527318, -3.143139765844555900 ) ) ;
#13959=CARTESIAN_POINT ( 'NONE',  ( 10.46874999795161720, 3.632567103900523620, 3.270778111535338262 ) ) ;
#13974=EDGE_CURVE ( 'NONE', #11016, #6403, #19351, .T. ) ;
#13976=DIRECTION ( 'NONE',  ( -0.000000000000000000, 0.000000000000000000, 1.000000000000000000 ) ) ;
#13993=ADVANCED_FACE ( 'NONE', ( #16265 ), #2357, .T. ) ;
#13994=LINE ( 'NONE', #18884, #9485 ) ;
#13995=ORIENTED_EDGE ( 'NONE', *, *, #17258, .F. ) ;
#13997=CARTESIAN_POINT ( 'NONE',  ( 10.34374999795161543, -4.150607464521772094, -2.695436003842760275 ) ) ;
#14009=CARTESIAN_POINT ( 'NONE',  ( 11.00000000000000711, 2.849999999999989431, 4.936344801571308061 ) ) ;
#14010=CARTESIAN_POINT ( 'NONE',  ( 13.00000000000000000, -3.840809689102975710, 4.211671987713753396 ) ) ;
#14015=CARTESIAN_POINT ( 'NONE',  ( 10.96874999795161720, -4.888101187500005551, 0.7741991708318548548 ) ) ;
#14032=EDGE_CURVE ( 'NONE', #15581, #6896, #16258, .T. ) ;
#14037=DIRECTION ( 'NONE',  ( -0.4999999999999980016, 0.7500000000000048850, -0.4330127018922129700 ) ) ;
#14039=VECTOR ( 'NONE', #9655, 1000.000000000000114 ) ;
#14056=CARTESIAN_POINT ( 'NONE',  ( 9.468749997951615427, 0.5109457054261445919, 4.861323657744411442 ) ) ;
#14058=EDGE_CURVE ( 'NONE', #6283, #14247, #5547, .T. ) ;
#14067=EDGE_LOOP ( 'NONE', ( #3213, #10918, #16562, #2000 ) ) ;
#14074=ORIENTED_EDGE ( 'NONE', *, *, #5985, .T. ) ;
#14078=CARTESIAN_POINT ( 'NONE',  ( 13.00000000000000178, 3.908719486245998187, -2.935207862669990231 ) ) ;
#14088=CARTESIAN_POINT ( 'NONE',  ( 13.00000000000000000, -4.125339889944092953, 2.622041954598548941 ) ) ;
#14092=CARTESIAN_POINT ( 'NONE',  ( 11.50000000000000355, 5.699999999999999289, 0.9027913098498566713 ) ) ;
#14097=EDGE_CURVE ( 'NONE', #15404, #7834, #9253, .T. ) ;
#14100=CYLINDRICAL_SURFACE ( 'NONE', #100, 5.700000000000001954 ) ;
#14101=AXIS2_PLACEMENT_3D ( 'NONE', #4735, #12545, #18732 ) ;
#14102=CARTESIAN_POINT ( 'NONE',  ( 6.968749997951614539, 4.620319390059829168, -1.773574444220725077 ) ) ;
#14110=CARTESIAN_POINT ( 'NONE',  ( 14.46874999795161720, -2.873153789725797935, -3.954556930911881096 ) ) ;
#14136=CARTESIAN_POINT ( 'NONE',  ( 7.078124996927420476, -4.584782303107616031, 2.647025296874957689 ) ) ;
#14154=DIRECTION ( 'NONE',  ( 0.000000000000000000, 0.000000000000000000, 1.000000000000000000 ) ) ;
#14155=CARTESIAN_POINT ( 'NONE',  ( 6.968749997951614539, 4.620319390059829168, -1.773574444220725077 ) ) ;
#14172=CARTESIAN_POINT ( 'NONE',  ( 13.00000000000000178, 0.7793280607715257213, 4.825575716215943167 ) ) ;
#14176=EDGE_LOOP ( 'NONE', ( #14074, #8107, #10526, #1973, #14671 ) ) ;
#14184=CARTESIAN_POINT ( 'NONE',  ( 14.34374999795161365, 4.780397808154273065, -1.280903732194386802 ) ) ;
#14193=EDGE_CURVE ( 'NONE', #9700, #7035, #14481, .T. ) ;
#14205=FACE_OUTER_BOUND ( 'NONE', #4882, .T. ) ;
#14207=CARTESIAN_POINT ( 'NONE',  ( 6.468749997951615427, -4.233219804643904460, 2.444050593749960587 ) ) ;
#14239=CARTESIAN_POINT ( 'NONE',  ( -0.000000000000000000, 0.000000000000000000, 0.000000000000000000 ) ) ;
#14247=VERTEX_POINT ( 'NONE', #8448 ) ;
#14253=ORIENTED_EDGE ( 'NONE', *, *, #8136, .F. ) ;
#14262=CARTESIAN_POINT ( 'NONE',  ( 10.46874999795161720, -1.016293382781444654, 4.781284448697187273 ) ) ;
#14271=CARTESIAN_POINT ( 'NONE',  ( 10.00000000000000533, -5.421022142882388373, 1.761396867937162769 ) ) ;
#14291=CARTESIAN_POINT ( 'NONE',  ( 11.00000000000000711, 5.700000000000001066, -3.490243377569957047E-16 ) ) ;
#14311=CARTESIAN_POINT ( 'NONE',  ( 10.34374999795161543, -4.409619785863921670, 2.246813503491803310 ) ) ;
#14316=DIRECTION ( 'NONE',  ( 1.000000000000000000, -0.000000000000000000, -0.000000000000000000 ) ) ;
#14321=CARTESIAN_POINT ( 'NONE',  ( 10.81249999590322375, 5.142044285764750811, -2.620002426024544473 ) ) ;
#14331=CARTESIAN_POINT ( 'NONE',  ( -2.000000000000001776, -3.218695387886217674, 2.999999999999999112 ) ) ;
#14359=( BOUNDED_CURVE ( )  B_SPLINE_CURVE ( 2, ( #496, #7983, #6569, #12697, #18791, #1081, #7156, #9906, #6965, #887, #17689, #4179, #12995, #5763, #13190 ),
 .UNSPECIFIED., .F., .F. ) 
 B_SPLINE_CURVE_WITH_KNOTS ( ( 3, 2, 2, 2, 2, 2, 2, 3 ),
 ( 0.000000000000000000, 0.05000000000000000278, 0.1000000000000000056, 0.1499999999999999944, 0.2000000000000000111, 0.2500000000000000000, 0.2999999999999999889, 0.3078686208676164604 ),
 .UNSPECIFIED. ) 
 CURVE ( )  GEOMETRIC_REPRESENTATION_ITEM ( )  RATIONAL_B_SPLINE_CURVE ( ( 1.000000000000000000, 0.9876883405951377704, 1.000000000000000000, 0.9876883405951377704, 1.000000000000000000, 0.9876883405951377704, 1.000000000000000000, 0.9876883405951377704, 1.000000000000000000, 0.9876883405951377704, 1.000000000000000000, 0.9876883405951377704, 1.000000000000000000, 0.9980624843978382899, 0.9967347918236166837 ) ) 
 REPRESENTATION_ITEM ( '' )  );
#14363=CARTESIAN_POINT ( 'NONE',  ( 6.968749997951614539, 3.846120219227923798, 3.114526743279282694 ) ) ;
#14371=CARTESIAN_POINT ( 'NONE',  ( 11.00000000000000711, -5.700000000000001066, -3.945386292505473391E-14 ) ) ;
#14382=B_SPLINE_CURVE_WITH_KNOTS ( 'NONE', 3,
 ( #12055, #1446, #18446, #9152 ),
 .UNSPECIFIED., .F., .F.,
 ( 4, 4 ),
 ( 0.000000000000000000, 0.001126652051248517921 ),
 .UNSPECIFIED. ) ;
#14387=EDGE_CURVE ( 'NONE', #16939, #18923, #19418, .T. ) ;
#14389=LINE ( 'NONE', #18682, #13800 ) ;
#14390=CARTESIAN_POINT ( 'NONE',  ( 11.34374999795161543, 1.773574444220789914, -4.620319390059805187 ) ) ;
#14408=CARTESIAN_POINT ( 'NONE',  ( 8.968749997951611874, -4.780397808154247308, -1.280903732194487166 ) ) ;
#14450=DIRECTION ( 'NONE',  ( 0.000000000000000000, 0.000000000000000000, -1.000000000000000000 ) ) ;
#14458=CARTESIAN_POINT ( 'NONE',  ( 13.00000000000000000, -5.567819778318897406, -1.220402768007724292 ) ) ;
#14465=CARTESIAN_POINT ( 'NONE',  ( 11.31249999590322375, -5.421022142882388373, 1.761396867937162769 ) ) ;
#14466=CARTESIAN_POINT ( 'NONE',  ( 12.73273607671833929, -3.906077990787160559, 2.967013497617006834 ) ) ;
#14470=EDGE_CURVE ( 'NONE', #2028, #3546, #5179, .T. ) ;
#14476=EDGE_CURVE ( 'NONE', #8156, #10630, #14359, .T. ) ;
#14480=CARTESIAN_POINT ( 'NONE',  ( 11.50000000000000355, -5.699999999999994849, -0.9027913098498963063 ) ) ;
#14481=( BOUNDED_CURVE ( )  B_SPLINE_CURVE ( 2, ( #6136, #6523, #16861, #3345, #12653, #13853, #9456, #15553, #18744, #5038, #11150, #17247, #15360, #8140, #146 ),
 .UNSPECIFIED., .F., .F. ) 
 B_SPLINE_CURVE_WITH_KNOTS ( ( 3, 2, 2, 2, 2, 2, 2, 3 ),
 ( 0.000000000000000000, 0.04999999999999999584, 0.09999999999999999167, 0.1499999999999999944, 0.1999999999999999833, 0.2500000000000000000, 0.2999999999999999889, 0.3499999999999999778 ),
 .UNSPECIFIED. ) 
 CURVE ( )  GEOMETRIC_REPRESENTATION_ITEM ( )  RATIONAL_B_SPLINE_CURVE ( ( 1.000000000000000000, 0.9876883405951377704, 1.000000000000000000, 0.9876883405951377704, 1.000000000000000000, 0.9876883405951377704, 1.000000000000000000, 0.9876883405951377704, 1.000000000000000000, 0.9876883405951377704, 1.000000000000000000, 0.9876883405951377704, 1.000000000000000000, 0.9876883405951377704, 1.000000000000000000 ) ) 
 REPRESENTATION_ITEM ( '' )  );
#14486=EDGE_CURVE ( 'NONE', #15, #18486, #16517, .T. ) ;
#14492=CARTESIAN_POINT ( 'NONE',  ( 13.00000000000000178, 3.830176896397430752, -3.037670790816736410 ) ) ;
#14496=CARTESIAN_POINT ( 'NONE',  ( 14.46874999795161720, 4.861323657744413218, -0.5109457054261112852 ) ) ;
#14511=EDGE_LOOP ( 'NONE', ( #5491, #5719, #19535, #16272 ) ) ;
#14515=CARTESIAN_POINT ( 'NONE',  ( 7.468749997951615427, -4.781284448697200595, 1.016293382781377819 ) ) ;
#14519=CARTESIAN_POINT ( 'NONE',  ( 14.81249999590322552, -4.080749450109621534, -4.080749450109677490 ) ) ;
#14528=DIRECTION ( 'NONE',  ( 0.000000000000000000, 0.8660254037844432595, -0.4999999999999920619 ) ) ;
#14535=CARTESIAN_POINT ( 'NONE',  ( 7.812499995903224637, -5.387740456496247887, 2.068159791354145849 ) ) ;
#14546=ORIENTED_EDGE ( 'NONE', *, *, #9084, .T. ) ;
#14591=CARTESIAN_POINT ( 'NONE',  ( 10.34374999795161543, 0.2590123213421660631, -4.942249507334554259 ) ) ;
#14600=CARTESIAN_POINT ( 'NONE',  ( 12.84374999795161543, -1.016293382781378485, -4.781284448697201483 ) ) ;
#14611=DIRECTION ( 'NONE',  ( 0.000000000000000000, -0.7315216790650492795, 0.6818181818181815457 ) ) ;
#14614=CARTESIAN_POINT ( 'NONE',  ( 6.843749997951615427, -3.413342815706642518E-14, 4.888101187500000222 ) ) ;
#14615=DIRECTION ( 'NONE',  ( 1.000000000000000000, 0.000000000000000000, 0.000000000000000000 ) ) ;
#14618=EDGE_CURVE ( 'NONE', #14637, #11664, #7658, .T. ) ;
#14621=CARTESIAN_POINT ( 'NONE',  ( 6.843749997951615427, 4.233219804643871598, 2.444050593750020095 ) ) ;
#14629=ORIENTED_EDGE ( 'NONE', *, *, #8678, .F. ) ;
#14637=VERTEX_POINT ( 'NONE', #10776 ) ;
#14658=ORIENTED_EDGE ( 'NONE', *, *, #16149, .T. ) ;
#14660=CARTESIAN_POINT ( 'NONE',  ( 13.00000000000000000, -5.567819778318897406, -1.220402768007724292 ) ) ;
#14671=ORIENTED_EDGE ( 'NONE', *, *, #17717, .T. ) ;
#14672=CARTESIAN_POINT ( 'NONE',  ( 7.468749997951615427, -4.781284448697200595, 1.016293382781377819 ) ) ;
#14682=CYLINDRICAL_SURFACE ( 'NONE', #10497, 5.700000000000001954 ) ;
#14687=CARTESIAN_POINT ( 'NONE',  ( 7.843749997951614539, -3.270778111535287191, -3.632567103900569361 ) ) ;
#14710=FACE_OUTER_BOUND ( 'NONE', #4118, .T. ) ;
#14714=ADVANCED_FACE ( 'NONE', ( #17178, #18767 ), #12774, .F. ) ;
#14723=AXIS2_PLACEMENT_3D ( 'NONE', #16521, #7595, #2896 ) ;
#14725=FACE_OUTER_BOUND ( 'NONE', #4517, .T. ) ;
#14730=CARTESIAN_POINT ( 'NONE',  ( -2.000000000000001776, 0.000000000000000000, 0.000000000000000000 ) ) ;
#14752=CARTESIAN_POINT ( 'NONE',  ( 13.50000000000000533, 1.493657965219562067, -5.574407415329146964 ) ) ;
#14754=CARTESIAN_POINT ( 'NONE',  ( 2.999999999999998224, 3.950217066951266176, 3.681818181818181213 ) ) ;
#14755=ORIENTED_EDGE ( 'NONE', *, *, #6322, .T. ) ;
#14759=CIRCLE ( 'NONE', #8686, 6.500000000000000000 ) ;
#14772=CARTESIAN_POINT ( 'NONE',  ( 6.500000000000005329, 4.484949146646356688, 3.631840208645826795 ) ) ;
#14780=CARTESIAN_POINT ( 'NONE',  ( 8.312499995903225525, -3.814044456245443193, -4.235925505221191933 ) ) ;
#14796=CIRCLE ( 'NONE', #6793, 4.400000000000000355 ) ;
#14798=LINE ( 'NONE', #19287, #4486 ) ;
#14806=ORIENTED_EDGE ( 'NONE', *, *, #1499, .T. ) ;
#14815=CARTESIAN_POINT ( 'NONE',  ( 7.312499995903225525, -3.980288726281172656E-14, 5.700000000000001066 ) ) ;
#14834=B_SPLINE_CURVE_WITH_KNOTS ( 'NONE', 3,
 ( #12684, #12783, #1876, #18775, #2169, #8376, #14078, #18880, #14492, #9893 ),
 .UNSPECIFIED., .F., .F.,
 ( 4, 3, 3, 4 ),
 ( 0.000000000000000000, 0.0001875345074742620726, 0.0003808595644229701067, 0.0005744879655065565855 ),
 .UNSPECIFIED. ) ;
#14838=CARTESIAN_POINT ( 'NONE',  ( 12.84374999795161543, -3.632567103900546712, 3.270778111535314281 ) ) ;
#14846=DIRECTION ( 'NONE',  ( -0.000000000000000000, -0.7315216790650492795, -0.6818181818181815457 ) ) ;
#14852=ORIENTED_EDGE ( 'NONE', *, *, #8769, .F. ) ;
#14853=EDGE_CURVE ( 'NONE', #13643, #11673, #12960, .T. ) ;
#14871=CARTESIAN_POINT ( 'NONE',  ( 8.500000000000007105, 1.493657965219485018, 5.574407415329170057 ) ) ;
#14878=SHAPE_REPRESENTATION ( 'CLUTCH CONE', ( #16724 ), #12592 ) ;
#14885=CARTESIAN_POINT ( 'NONE',  ( 12.81249999590322552, 5.699999999999999289, 0.9027913098498566713 ) ) ;
#14886=CARTESIAN_POINT ( 'NONE',  ( 10.84374999795161543, -3.632567103900500971, -3.270778111535363131 ) ) ;
#14890=SHAPE_REPRESENTATION_RELATIONSHIP ( 'NONE' , 'NONE' ,  #14878, #7808 ) ;
#14894=CARTESIAN_POINT ( 'NONE',  ( 2.999999999999998224, 0.000000000000000000, 0.000000000000000000 ) ) ;
#14919=CARTESIAN_POINT ( 'NONE',  ( 10.46874999795161720, 4.648860486681953397, -1.510506337161861667 ) ) ;
#14944=CARTESIAN_POINT ( 'NONE',  ( 13.46874999795161543, 0.5109457054262118714, -4.861323657744403448 ) ) ;
#14946=LINE ( 'NONE', #2631, #2159 ) ;
#14960=DIRECTION ( 'NONE',  ( 0.000000000000000000, 0.000000000000000000, 1.000000000000000000 ) ) ;
#14994=( BOUNDED_CURVE ( )  B_SPLINE_CURVE ( 2, ( #13232, #17539, #1217, #5610, #6910, #19514, #16232 ),
 .UNSPECIFIED., .F., .F. ) 
 B_SPLINE_CURVE_WITH_KNOTS ( ( 3, 2, 2, 3 ),
 ( 0.1666819079834116757, 0.2000000000000000111, 0.2500000000000000000, 0.2843253191101273170 ),
 .UNSPECIFIED. ) 
 CURVE ( )  GEOMETRIC_REPRESENTATION_ITEM ( )  RATIONAL_B_SPLINE_CURVE ( ( 0.9945256517182512468, 0.9917959799814380917, 1.000000000000000000, 0.9876883405951377704, 1.000000000000000000, 0.9915479672430580482, 0.9947006833465674713 ) ) 
 REPRESENTATION_ITEM ( '' )  );
#14996=CARTESIAN_POINT ( 'NONE',  ( 6.468749997951615427, 0.000000000000000000, -4.888101187500000222 ) ) ;
#15002=CARTESIAN_POINT ( 'NONE',  ( 14.81249999590322552, -5.574407415329169169, 1.493657965219485462 ) ) ;
#15006=CARTESIAN_POINT ( 'NONE',  ( -2.000000000000001776, 0.000000000000000000, 0.000000000000000000 ) ) ;
#15009=CARTESIAN_POINT ( 'NONE',  ( 10.96874999795161720, 4.888101187500000222, -0.7741991708318890497 ) ) ;
#15012=CARTESIAN_POINT ( 'NONE',  ( 13.50000000000000533, -4.080749450109621534, -4.080749450109677490 ) ) ;
#15027=FACE_OUTER_BOUND ( 'NONE', #4404, .T. ) ;
#15036=CARTESIAN_POINT ( 'NONE',  ( -2.000000000000001776, 0.000000000000000000, 4.400000000000000355 ) ) ;
#15075=EDGE_CURVE ( 'NONE', #7035, #11673, #5863, .T. ) ;
#15083=CARTESIAN_POINT ( 'NONE',  ( 13.34374999795161365, 4.409619785863906571, 2.246813503491833508 ) ) ;
#15094=VECTOR ( 'NONE', #10498, 1000.000000000000000 ) ;
#15102=CARTESIAN_POINT ( 'NONE',  ( 7.312499995903225525, 4.936344801571289409, 2.850000000000024070 ) ) ;
#15103=CARTESIAN_POINT ( 'NONE',  ( 7.812499995903224637, -5.387740456496247887, 2.068159791354145849 ) ) ;
#15107=CARTESIAN_POINT ( 'NONE',  ( 11.00000000000000711, 2.849999999999989431, 4.936344801571308061 ) ) ;
#15117=CARTESIAN_POINT ( 'NONE',  ( 7.468749997951615427, -1.510506337161893864, 4.648860486681943627 ) ) ;
#15127=ADVANCED_FACE ( 'NONE', ( #4844 ), #343, .F. ) ;
#15137=CARTESIAN_POINT ( 'NONE',  ( 5.500000000000005329, 0.000000000000000000, 0.000000000000000000 ) ) ;
#15143=CARTESIAN_POINT ( 'NONE',  ( 6.500000000000005329, -5.387740456496247887, 2.068159791354145849 ) ) ;
#15144=CARTESIAN_POINT ( 'NONE',  ( 13.00000000000000178, 0.6516788101670740740, 4.844895625238696546 ) ) ;
#15146=CARTESIAN_POINT ( 'NONE',  ( 13.00000000000000533, -4.859449410165145977, 2.460251518383743896 ) ) ;
#15168=VECTOR ( 'NONE', #9531, 1000.000000000000000 ) ;
#15180=CARTESIAN_POINT ( 'NONE',  ( 14.31249999590322552, 4.611396867937201272, 3.350375938067096548 ) ) ;
#15202=CARTESIAN_POINT ( 'NONE',  ( 8.812499995903225525, 3.143139765844590983, 4.840010801796506890 ) ) ;
#15205=CARTESIAN_POINT ( 'NONE',  ( 13.31249999590322730, -1.185096637661177343, -5.575441324182703440 ) ) ;
#15209=CARTESIAN_POINT ( 'NONE',  ( 7.500000000000005329, 5.763142191869157216, -0.3020334839682475847 ) ) ;
#15211=CARTESIAN_POINT ( 'NONE',  ( 6.468749997951615427, 0.000000000000000000, -4.888101187500000222 ) ) ;
#15217=CARTESIAN_POINT ( 'NONE',  ( 13.84374999795161543, -4.465502636338038123, 1.988169868018562880 ) ) ;
#15218=CARTESIAN_POINT ( 'NONE',  ( 12.73273607671833929, -4.522548057701222923, -1.899256020376466569 ) ) ;
#15219=CARTESIAN_POINT ( 'NONE',  ( 10.96874999795161720, 4.888101187500000222, -0.7741991708318890497 ) ) ;
#15236=CARTESIAN_POINT ( 'NONE',  ( 8.312499995903225525, 5.575441324182696334, -1.185096637661215535 ) ) ;
#15248=CARTESIAN_POINT ( 'NONE',  ( -0.000000000000000000, 0.000000000000000000, 0.000000000000000000 ) ) ;
#15253=B_SPLINE_CURVE_WITH_KNOTS ( 'NONE', 3,
 ( #19509, #16525, #2803, #5798 ),
 .UNSPECIFIED., .F., .F.,
 ( 4, 4 ),
 ( 0.000000000000000000, 0.001125480700308659470 ),
 .UNSPECIFIED. ) ;
#15306=CARTESIAN_POINT ( 'NONE',  ( 9.312499995903225525, -5.668774803599153422, -0.5958122406256771697 ) ) ;
#15307=VECTOR ( 'NONE', #6836, 1000.000000000000000 ) ;
#15316=CARTESIAN_POINT ( 'NONE',  ( 10.46874999795161720, -1.016293382781444654, 4.781284448697187273 ) ) ;
#15326=CARTESIAN_POINT ( 'NONE',  ( 9.468749997951615427, -3.954556930911881985, 2.873153789725797491 ) ) ;
#15330=CARTESIAN_POINT ( 'NONE',  ( 12.50000000000000533, 4.840010801796527318, -3.143139765844555900 ) ) ;
#15349=CARTESIAN_POINT ( 'NONE',  ( 10.46874999795161720, 3.632567103900523620, 3.270778111535338262 ) ) ;
#15360=CARTESIAN_POINT ( 'NONE',  ( 12.00000000000000533, -1.185096637661177343, -5.575441324182703440 ) ) ;
#15372=CARTESIAN_POINT ( 'NONE',  ( 13.00000000000000178, 4.568735188514060575, 1.737869959597756697 ) ) ;
#15375=LINE ( 'NONE', #10675, #9989 ) ;
#15380=CARTESIAN_POINT ( 'NONE',  ( 13.00000000000000000, -0.2080849974988778772, -4.883670121236158401 ) ) ;
#15397=CARTESIAN_POINT ( 'NONE',  ( 13.00000000000000178, -4.568735188514048140, -1.737869959597788672 ) ) ;
#15404=VERTEX_POINT ( 'NONE', #13332 ) ;
#15407=CARTESIAN_POINT ( 'NONE',  ( 9.000000000000005329, 4.611396867937201272, -3.350375938067097437 ) ) ;
#15414=VECTOR ( 'NONE', #9484, 1000.000000000000000 ) ;
#15420=CARTESIAN_POINT ( 'NONE',  ( 5.500000000000005329, 0.000000000000000000, -32.79058411375427795 ) ) ;
#15421=EDGE_CURVE ( 'NONE', #16744, #11644, #8933, .T. ) ;
#15445=CARTESIAN_POINT ( 'NONE',  ( 11.46874999795161543, 2.444050593749990785, 4.233219804643887585 ) ) ;
#15450=DIRECTION ( 'NONE',  ( 1.000000000000000000, -0.000000000000000000, -0.000000000000000000 ) ) ;
#15460=ORIENTED_EDGE ( 'NONE', *, *, #4889, .T. ) ;
#15461=CARTESIAN_POINT ( 'NONE',  ( 12.99999999999998401, 0.02830770314434387022, -5.175540411820488629 ) ) ;
#15465=CARTESIAN_POINT ( 'NONE',  ( 7.468749997951615427, 4.781284448697194378, -1.016293382781411125 ) ) ;
#15477=CARTESIAN_POINT ( 'NONE',  ( 11.96874999795161365, -1.773574444220693325, -4.620319390059841602 ) ) ;
#15479=CARTESIAN_POINT ( 'NONE',  ( 13.00000000000000178, -0.5236311934647339683, -4.860400829920959787 ) ) ;
#15487=ORIENTED_EDGE ( 'NONE', *, *, #8136, .T. ) ;
#15499=CARTESIAN_POINT ( 'NONE',  ( 6.000000000000005329, -4.936344801571268093, -2.850000000000058265 ) ) ;
#15513=CARTESIAN_POINT ( 'NONE',  ( 8.000000000000005329, 5.668774803599156975, 0.5958122406256382009 ) ) ;
#15515=ORIENTED_EDGE ( 'NONE', *, *, #6539, .T. ) ;
#15525=( BOUNDED_SURFACE ( )  B_SPLINE_SURFACE ( 1, 2, ( 
 ( #9105, #15103, #2685, #5782, #15306, #12001, #7373, #4198, #7175, #10311, #19494, #13396, #15205, #7581, #16408, #10408, #13495 ),
 ( #16508, #18106, #6081, #7785, #12599, #18397, #1786, #13997, #17003, #1884, #7978, #18787, #10993, #91, #6276, #7682, #12495 ) ),
 .UNSPECIFIED., .F., .F., .T. ) 
 B_SPLINE_SURFACE_WITH_KNOTS ( ( 2, 2 ),
 ( 3, 2, 2, 2, 2, 2, 2, 2, 3 ),
 ( 0.000000000000000000, 1.000000000000000000 ),
 ( 0.000000000000000000, 0.05000000000000000278, 0.1000000000000000056, 0.1499999999999999944, 0.2000000000000000111, 0.2500000000000000000, 0.2999999999999999889, 0.3499999999999999778, 0.4000000000000000222 ),
 .UNSPECIFIED. ) 
 GEOMETRIC_REPRESENTATION_ITEM ( )  RATIONAL_B_SPLINE_SURFACE ( (
 ( 1.000000000000000000, 0.9876883405951377704, 1.000000000000000000, 0.9876883405951377704, 1.000000000000000000, 0.9876883405951377704, 1.000000000000000000, 0.9876883405951377704, 1.000000000000000000, 0.9876883405951377704, 1.000000000000000000, 0.9876883405951377704, 1.000000000000000000, 0.9876883405951377704, 1.000000000000000000, 0.9876883405951377704, 1.000000000000000000),
 ( 1.000000000000000000, 0.9876883405951377704, 1.000000000000000000, 0.9876883405951377704, 1.000000000000000000, 0.9876883405951377704, 1.000000000000000000, 0.9876883405951377704, 1.000000000000000000, 0.9876883405951377704, 1.000000000000000000, 0.9876883405951377704, 1.000000000000000000, 0.9876883405951377704, 1.000000000000000000, 0.9876883405951377704, 1.000000000000000000) ) ) 
 REPRESENTATION_ITEM ( '' )  SURFACE ( )  );
#15548=VERTEX_POINT ( 'NONE', #9234 ) ;
#15553=CARTESIAN_POINT ( 'NONE',  ( 9.500000000000005329, -4.840010801796461593, -3.143139765844656264 ) ) ;
#15560=CARTESIAN_POINT ( 'NONE',  ( 13.96874999795161365, -1.280903732194453859, 4.780397808154257078 ) ) ;
#15573=CARTESIAN_POINT ( 'NONE',  ( 13.96874999795161365, 1.280903732194486722, -4.780397808154247308 ) ) ;
#15581=VERTEX_POINT ( 'NONE', #5504 ) ;
#15593=CARTESIAN_POINT ( 'NONE',  ( 12.92161831991541554, -4.611601942845651614, -1.625176344145968788 ) ) ;
#15600=DIRECTION ( 'NONE',  ( 0.000000000000000000, -0.7315216790650493905, 0.6818181818181815457 ) ) ;
#15610=CARTESIAN_POINT ( 'NONE',  ( 13.46874999795161543, -0.5109457054261780096, 4.861323657744406113 ) ) ;
#15617=CARTESIAN_POINT ( 'NONE',  ( 13.46874999795161543, -3.954556930911842016, -2.873153789725852558 ) ) ;
#15626=ORIENTED_EDGE ( 'NONE', *, *, #11729, .F. ) ;
#15659=CARTESIAN_POINT ( 'NONE',  ( 8.968749997951611874, 4.780397808154257078, 1.280903732194454303 ) ) ;
#15671=CARTESIAN_POINT ( 'NONE',  ( 14.46874999795161720, 1.988169868018623720, -4.465502636338010589 ) ) ;
#15676=CARTESIAN_POINT ( 'NONE',  ( 13.00000000000000178, 1.070668164103456110, 5.063333171156721768 ) ) ;
#15687=CARTESIAN_POINT ( 'NONE',  ( 7.312499995903225525, -4.936344801571268093, -2.850000000000058265 ) ) ;
#15690=CARTESIAN_POINT ( 'NONE',  ( 11.00000000000000711, 2.850000000000057820, -4.936344801571268093 ) ) ;
#15718=TOROIDAL_SURFACE ( 'NONE', #7064, -32.79058411375427795, 40.00000000000000711 ) ;
#15721=CARTESIAN_POINT ( 'NONE',  ( 9.312499995903225525, 3.350375938067097437, -4.611396867937201272 ) ) ;
#15733=ADVANCED_FACE ( 'NONE', ( #12825 ), #9098, .F. ) ;
#15735=B_SPLINE_CURVE_WITH_KNOTS ( 'NONE', 3,
 ( #5052, #17464, #15964, #4958 ),
 .UNSPECIFIED., .F., .F.,
 ( 4, 4 ),
 ( 0.000000000000000000, 0.001126652051248517271 ),
 .UNSPECIFIED. ) ;
#15737=AXIS2_PLACEMENT_3D ( 'NONE', #289, #9599, #494 ) ;
#15744=ORIENTED_EDGE ( 'NONE', *, *, #8, .F. ) ;
#15757=CARTESIAN_POINT ( 'NONE',  ( 13.00000000000000533, 0.5958122406256767256, -5.668774803599153422 ) ) ;
#15761=CARTESIAN_POINT ( 'NONE',  ( 7.843749997951614539, 3.270778111535313837, 3.632567103900546712 ) ) ;
#15762=CARTESIAN_POINT ( 'NONE',  ( 12.34374999795161543, 1.773574444220725299, 4.620319390059829168 ) ) ;
#15777=ORIENTED_EDGE ( 'NONE', *, *, #6277, .T. ) ;
#15788=DIRECTION ( 'NONE',  ( -0.4999999999999978351, 0.7499999999999990008, 0.4330127018922234616 ) ) ;
#15790=DIRECTION ( 'NONE',  ( -1.000000000000000000, -0.000000000000000000, -0.000000000000000000 ) ) ;
#15798=CARTESIAN_POINT ( 'NONE',  ( 8.312499995903225525, 3.814044456245473835, 4.235925505221166176 ) ) ;
#15806=CARTESIAN_POINT ( 'NONE',  ( 13.00000000000000178, -3.789407127742538517, 3.087705756618167374 ) ) ;
#15814=EDGE_CURVE ( 'NONE', #5327, #12828, #664, .T. ) ;
#15815=CARTESIAN_POINT ( 'NONE',  ( 13.81249999590322552, -5.142044285764733935, -2.620002426024580000 ) ) ;
#15821=CARTESIAN_POINT ( 'NONE',  ( 13.00000000000000178, -0.7793280607714923036, -4.825575716215948496 ) ) ;
#15840=ORIENTED_EDGE ( 'NONE', *, *, #17523, .T. ) ;
#15861=CARTESIAN_POINT ( 'NONE',  ( 7.843749997951614539, 4.781284448697194378, -1.016293382781411125 ) ) ;
#15865=CARTESIAN_POINT ( 'NONE',  ( 7.812499995903224637, -0.9027913098498966393, 5.699999999999994849 ) ) ;
#15869=CIRCLE ( 'NONE', #11382, 5.400000000000000355 ) ;
#15890=CARTESIAN_POINT ( 'NONE',  ( 9.343749997951615427, -1.280903732194386579, -4.780397808154273953 ) ) ;
#15900=CARTESIAN_POINT ( 'NONE',  ( 8.812499995903225525, 3.143139765844590983, 4.840010801796506001 ) ) ;
#15909=CARTESIAN_POINT ( 'NONE',  ( 7.843749997951614539, -4.781284448697200595, 1.016293382781377819 ) ) ;
#15914=CARTESIAN_POINT ( 'NONE',  ( 12.84374999795161543, -4.648860486681943627, -1.510506337161893642 ) ) ;
#15921=DIRECTION ( 'NONE',  ( -0.4999999999999979461, -0.7500000000000021094, 0.4330127018922180770 ) ) ;
#15928=CARTESIAN_POINT ( 'NONE',  ( 12.46874999795161543, -4.648860486681943627, -1.510506337161893642 ) ) ;
#15964=CARTESIAN_POINT ( 'NONE',  ( 12.99999999999969980, -1.390454305316078276, -5.264438301130803133 ) ) ;
#15984=CARTESIAN_POINT ( 'NONE',  ( 7.468749997951615427, -3.270778111535287191, -3.632567103900569361 ) ) ;
#15985=CARTESIAN_POINT ( 'NONE',  ( 13.00000000000000533, -4.021726346896400628, 2.778353902928540453 ) ) ;
#16002=CARTESIAN_POINT ( 'NONE',  ( 8.468749997951615427, -4.861323657744403448, -0.5109457054262123155 ) ) ;
#16007=CARTESIAN_POINT ( 'NONE',  ( -2.000000000000001776, 3.478305785123968707, -3.241971077674649315 ) ) ;
#16015=CARTESIAN_POINT ( 'NONE',  ( 5.500000000000005329, -4.015688387708123076E-15, 32.79058411375427795 ) ) ;
#16032=LINE ( 'NONE', #16229, #3133 ) ;
#16033=ORIENTED_EDGE ( 'NONE', *, *, #12376, .F. ) ;
#16036=ADVANCED_FACE ( 'NONE', ( #9162 ), #5947, .T. ) ;
#16041=EDGE_CURVE ( 'NONE', #14247, #16782, #10665, .T. ) ;
#16045=ORIENTED_EDGE ( 'NONE', *, *, #14193, .F. ) ;
#16058=AXIS2_PLACEMENT_3D ( 'NONE', #18003, #5580, #16206 ) ;
#16062=CARTESIAN_POINT ( 'NONE',  ( 7.500000000000005329, 3.143139765844590983, 4.840010801796506001 ) ) ;
#16082=ORIENTED_EDGE ( 'NONE', *, *, #8120, .T. ) ;
#16091=CARTESIAN_POINT ( 'NONE',  ( 9.843749997951615427, -0.5109457054261099529, -4.861323657744413218 ) ) ;
#16093=CARTESIAN_POINT ( 'NONE',  ( 10.81249999590322375, 0.3020334839683282424, -5.763142191869152775 ) ) ;
#16111=CARTESIAN_POINT ( 'NONE',  ( 7.968749997951616315, -4.942249507334558700, 0.2590123213420631454 ) ) ;
#16117=CARTESIAN_POINT ( 'NONE',  ( 14.84374999795161543, -2.873153789725797935, -3.954556930911881096 ) ) ;
#16122=EDGE_CURVE ( 'NONE', #9700, #9124, #7002, .T. ) ;
#16123=AXIS2_PLACEMENT_3D ( 'NONE', #976, #18992, #17590 ) ;
#16127=ORIENTED_EDGE ( 'NONE', *, *, #4044, .T. ) ;
#16143=ORIENTED_EDGE ( 'NONE', *, *, #1665, .F. ) ;
#16147=ADVANCED_FACE ( 'NONE', ( #560 ), #17269, .F. ) ;
#16149=EDGE_CURVE ( 'NONE', #9454, #11016, #10851, .T. ) ;
#16154=FACE_OUTER_BOUND ( 'NONE', #3756, .T. ) ;
#16175=CARTESIAN_POINT ( 'NONE',  ( 8.000000000000005329, -3.350375938067129855, 4.611396867937178179 ) ) ;
#16191=EDGE_CURVE ( 'NONE', #15404, #13931, #5533, .T. ) ;
#16192=CARTESIAN_POINT ( 'NONE',  ( 13.00000000000000000, 3.840809689103004576, -4.211671987713725862 ) ) ;
#16202=CARTESIAN_POINT ( 'NONE',  ( 10.31249999590322552, 5.207209108562820710, 2.318398865532073749 ) ) ;
#16206=DIRECTION ( 'NONE',  ( 0.000000000000000000, -0.8660254037844398178, 0.4999999999999978351 ) ) ;
#16228=CARTESIAN_POINT ( 'NONE',  ( 13.00000000000000000, 5.567819778318904511, 1.220402768007685657 ) ) ;
#16229=CARTESIAN_POINT ( 'NONE',  ( 2.999999999999998224, 3.950217066951266176, -3.681818181818181213 ) ) ;
#16232=CARTESIAN_POINT ( 'NONE',  ( 13.00000000000000000, -3.840809689102975710, 4.211671987713753396 ) ) ;
#16250=DIRECTION ( 'NONE',  ( -1.000000000000000000, -0.000000000000000000, -0.000000000000000000 ) ) ;
#16253=CARTESIAN_POINT ( 'NONE',  ( 9.312499995903225525, -3.350375938067129855, 4.611396867937178179 ) ) ;
#16258=B_SPLINE_CURVE_WITH_KNOTS ( 'NONE', 3,
 ( #12868, #19062, #13065, #7033 ),
 .UNSPECIFIED., .F., .F.,
 ( 4, 4 ),
 ( 0.000000000000000000, 0.001125480700308659253 ),
 .UNSPECIFIED. ) ;
#16265=FACE_OUTER_BOUND ( 'NONE', #19402, .T. ) ;
#16267=LINE ( 'NONE', #3960, #5200 ) ;
#16272=ORIENTED_EDGE ( 'NONE', *, *, #7104, .F. ) ;
#16282=CARTESIAN_POINT ( 'NONE',  ( 13.00000000000000178, -3.947414994554141021, 2.883678330714922300 ) ) ;
#16289=CARTESIAN_POINT ( 'NONE',  ( 9.843749997951615427, -4.465502636338009701, -1.988169868018624609 ) ) ;
#16313=CARTESIAN_POINT ( 'NONE',  ( 6.968749997951614539, 0.7741991708318887166, -4.888101187500000222 ) ) ;
#16316=CARTESIAN_POINT ( 'NONE',  ( 8.500000000000007105, -4.080749450109678378, 4.080749450109621534 ) ) ;
#16335=CARTESIAN_POINT ( 'NONE',  ( 10.84374999795161543, 3.632567103900524064, 3.270778111535338262 ) ) ;
#16338=ORIENTED_EDGE ( 'NONE', *, *, #16122, .F. ) ;
#16341=CARTESIAN_POINT ( 'NONE',  ( -2.000000000000001776, -3.218695387886215453, -3.000000000000001776 ) ) ;
#16343=CARTESIAN_POINT ( 'NONE',  ( 2.999999999999998224, -3.950217066951263956, -3.681818181818183877 ) ) ;
#16350=EDGE_CURVE ( 'NONE', #9124, #1853, #8841, .T. ) ;
#16352=VECTOR ( 'NONE', #19149, 1000.000000000000000 ) ;
#16384=CARTESIAN_POINT ( 'NONE',  ( 8.343749997951611874, 2.246813503491833508, -4.409619785863906571 ) ) ;
#16399=( BOUNDED_SURFACE ( )  B_SPLINE_SURFACE ( 1, 2, ( 
 ( #5197, #5302, #12714, #6586, #9920, #19102, #9823, #6687, #17311, #3606, #11410, #5486, #9727, #15815, #17510, #14519, #2393 ),
 ( #14614, #8206, #11316, #6882, #3896, #902, #2101, #14311, #17418, #5396, #19196, #8409, #15914, #10019, #2195, #8303, #16117 ) ),
 .UNSPECIFIED., .F., .F., .F. ) 
 B_SPLINE_SURFACE_WITH_KNOTS ( ( 2, 2 ),
 ( 3, 2, 2, 2, 2, 2, 2, 2, 3 ),
 ( 0.000000000000000000, 1.000000000000000000 ),
 ( 0.000000000000000000, 0.05000000000000000278, 0.1000000000000000056, 0.1499999999999999944, 0.2000000000000000111, 0.2500000000000000000, 0.2999999999999999889, 0.3499999999999999778, 0.4000000000000000222 ),
 .UNSPECIFIED. ) 
 GEOMETRIC_REPRESENTATION_ITEM ( )  RATIONAL_B_SPLINE_SURFACE ( (
 ( 1.000000000000000000, 0.9876883405951377704, 1.000000000000000000, 0.9876883405951377704, 1.000000000000000000, 0.9876883405951377704, 1.000000000000000000, 0.9876883405951377704, 1.000000000000000000, 0.9876883405951377704, 1.000000000000000000, 0.9876883405951377704, 1.000000000000000000, 0.9876883405951377704, 1.000000000000000000, 0.9876883405951377704, 1.000000000000000000),
 ( 1.000000000000000000, 0.9876883405951377704, 1.000000000000000000, 0.9876883405951377704, 1.000000000000000000, 0.9876883405951377704, 1.000000000000000000, 0.9876883405951377704, 1.000000000000000000, 0.9876883405951377704, 1.000000000000000000, 0.9876883405951377704, 1.000000000000000000, 0.9876883405951377704, 1.000000000000000000, 0.9876883405951377704, 1.000000000000000000) ) ) 
 REPRESENTATION_ITEM ( '' )  SURFACE ( )  );
#16401=CARTESIAN_POINT ( 'NONE',  ( 6.656249997951614539, -4.936344801571268093, -2.850000000000058265 ) ) ;
#16407=CARTESIAN_POINT ( 'NONE',  ( 8.468749997951615427, -1.988169868018530462, -4.465502636338051445 ) ) ;
#16408=CARTESIAN_POINT ( 'NONE',  ( 14.31249999590322552, 0.5958122406256767256, -5.668774803599153422 ) ) ;
#16413=VERTEX_POINT ( 'NONE', #5022 ) ;
#16423=CARTESIAN_POINT ( 'NONE',  ( 6.468749997951615427, 0.000000000000000000, -4.888101187500000222 ) ) ;
#16440=CARTESIAN_POINT ( 'NONE',  ( 13.00000000000000178, 0.7793280607715257213, 4.825575716215943167 ) ) ;
#16452=CARTESIAN_POINT ( 'NONE',  ( 12.50000000000000533, -0.3020334839682081163, -5.763142191869158992 ) ) ;
#16456=CARTESIAN_POINT ( 'NONE',  ( 13.00000000000000000, -4.125339889944092953, 2.622041954598548941 ) ) ;
#16489=CARTESIAN_POINT ( 'NONE',  ( 10.34374999795161543, 4.409619785863906571, -2.246813503491833508 ) ) ;
#16492=SURFACE_STYLE_USAGE ( .BOTH. , #12285 ) ;
#16493=CARTESIAN_POINT ( 'NONE',  ( 6.000000000000005329, 0.000000000000000000, 0.000000000000000000 ) ) ;
#16495=ORIENTED_EDGE ( 'NONE', *, *, #979, .F. ) ;
#16506=CARTESIAN_POINT ( 'NONE',  ( 7.812499995903224637, 4.484949146646356688, 3.631840208645826795 ) ) ;
#16508=CARTESIAN_POINT ( 'NONE',  ( 6.843749997951615427, -4.233219804643904460, 2.444050593749960587 ) ) ;
#16513=CARTESIAN_POINT ( 'NONE',  ( 9.468749997951615427, 3.954556930911862000, -2.873153789725825469 ) ) ;
#16517=( BOUNDED_CURVE ( )  B_SPLINE_CURVE ( 2, ( #19086, #10096, #19279, #4083, #10188, #5473, #16289, #794, #14886, #5377, #19180, #11585, #14600, #17884, #17788 ),
 .UNSPECIFIED., .F., .F. ) 
 B_SPLINE_CURVE_WITH_KNOTS ( ( 3, 2, 2, 2, 2, 2, 2, 3 ),
 ( 0.000000000000000000, 0.05000000000000000278, 0.1000000000000000056, 0.1499999999999999944, 0.2000000000000000111, 0.2500000000000000000, 0.2999999999999999889, 0.3078686208676164604 ),
 .UNSPECIFIED. ) 
 CURVE ( )  GEOMETRIC_REPRESENTATION_ITEM ( )  RATIONAL_B_SPLINE_CURVE ( ( 1.000000000000000000, 0.9876883405951377704, 1.000000000000000000, 0.9876883405951377704, 1.000000000000000000, 0.9876883405951377704, 1.000000000000000000, 0.9876883405951377704, 1.000000000000000000, 0.9876883405951377704, 1.000000000000000000, 0.9876883405951377704, 1.000000000000000000, 0.9980624843978382899, 0.9967347918236166837 ) ) 
 REPRESENTATION_ITEM ( '' )  );
#16521=CARTESIAN_POINT ( 'NONE',  ( -0.000000000000000000, 0.000000000000000000, 0.000000000000000000 ) ) ;
#16524=CARTESIAN_POINT ( 'NONE',  ( 13.00000000000000178, 0.000000000000000000, 0.000000000000000000 ) ) ;
#16525=CARTESIAN_POINT ( 'NONE',  ( 13.00000000000000533, -4.560365019702126155, -2.978280878416461164 ) ) ;
#16540=CARTESIAN_POINT ( 'NONE',  ( 12.46874999795161543, 4.648860486681953397, 1.510506337161861223 ) ) ;
#16553=AXIS2_PLACEMENT_3D ( 'NONE', #1312, #7389, #4410 ) ;
#16562=ORIENTED_EDGE ( 'NONE', *, *, #5520, .T. ) ;
#16568=CARTESIAN_POINT ( 'NONE',  ( 10.46874999795161720, -3.632567103900500971, -3.270778111535363131 ) ) ;
#16572=VERTEX_POINT ( 'NONE', #14331 ) ;
#16585=CARTESIAN_POINT ( 'NONE',  ( 12.31249999590322552, 5.700000000000001066, -3.490243377569957047E-16 ) ) ;
#16597=CARTESIAN_POINT ( 'NONE',  ( 12.99999999999999467, 4.444590484536241171, 2.035510078342908091 ) ) ;
#16604=CARTESIAN_POINT ( 'NONE',  ( 9.812499995903223748, 1.493657965219485018, 5.574407415329170057 ) ) ;
#16606=CARTESIAN_POINT ( 'NONE',  ( 9.468749997951615427, -0.5109457054261099529, -4.861323657744413218 ) ) ;
#16607=DIRECTION ( 'NONE',  ( 0.000000000000000000, 0.000000000000000000, 1.000000000000000000 ) ) ;
#16611=CARTESIAN_POINT ( 'NONE',  ( 8.000000000000005329, -3.350375938067129855, 4.611396867937178179 ) ) ;
#16614=CARTESIAN_POINT ( 'NONE',  ( 8.468749997951615427, -2.873153789725853002, 3.954556930911842016 ) ) ;
#16615=CARTESIAN_POINT ( 'NONE',  ( 7.968749997951616315, 2.246813503491833508, -4.409619785863906571 ) ) ;
#16622=PLANE ( 'NONE',  #7707 ) ;
#16627=( BOUNDED_SURFACE ( )  B_SPLINE_SURFACE ( 1, 2, ( 
 ( #13614, #19414, #4500, #7597, #5796, #1309, #16722, #11917, #10617, #10329, #13511, #3103, #1211, #19782, #7288, #3002, #9116 ),
 ( #16423, #11815, #7494, #16615, #13408, #17922, #4311, #2700, #14919, #15219, #18029, #19712, #1513, #13713, #10422, #5996, #7387 ) ),
 .UNSPECIFIED., .F., .F., .F. ) 
 B_SPLINE_SURFACE_WITH_KNOTS ( ( 2, 2 ),
 ( 3, 2, 2, 2, 2, 2, 2, 2, 3 ),
 ( 0.000000000000000000, 1.000000000000000000 ),
 ( 0.000000000000000000, 0.05000000000000000278, 0.1000000000000000056, 0.1499999999999999944, 0.2000000000000000111, 0.2500000000000000000, 0.2999999999999999889, 0.3499999999999999778, 0.4000000000000000222 ),
 .UNSPECIFIED. ) 
 GEOMETRIC_REPRESENTATION_ITEM ( )  RATIONAL_B_SPLINE_SURFACE ( (
 ( 1.000000000000000000, 0.9876883405951377704, 1.000000000000000000, 0.9876883405951377704, 1.000000000000000000, 0.9876883405951377704, 1.000000000000000000, 0.9876883405951377704, 1.000000000000000000, 0.9876883405951377704, 1.000000000000000000, 0.9876883405951377704, 1.000000000000000000, 0.9876883405951377704, 1.000000000000000000, 0.9876883405951377704, 1.000000000000000000),
 ( 1.000000000000000000, 0.9876883405951377704, 1.000000000000000000, 0.9876883405951377704, 1.000000000000000000, 0.9876883405951377704, 1.000000000000000000, 0.9876883405951377704, 1.000000000000000000, 0.9876883405951377704, 1.000000000000000000, 0.9876883405951377704, 1.000000000000000000, 0.9876883405951377704, 1.000000000000000000, 0.9876883405951377704, 1.000000000000000000) ) ) 
 REPRESENTATION_ITEM ( '' )  SURFACE ( )  );
#16630=CARTESIAN_POINT ( 'NONE',  ( 12.99999999999998757, 4.496303326521696064, -2.563255015864441155 ) ) ;
#16631=CARTESIAN_POINT ( 'NONE',  ( 7.312499995903225525, 4.936344801571308061, -2.849999999999989431 ) ) ;
#16634=ORIENTED_EDGE ( 'NONE', *, *, #18771, .F. ) ;
#16641=DIRECTION ( 'NONE',  ( 1.000000000000000000, 0.000000000000000000, 0.000000000000000000 ) ) ;
#16645=CARTESIAN_POINT ( 'NONE',  ( 7.968749997951616315, 4.942249507334556924, -0.2590123213420971182 ) ) ;
#16648=ADVANCED_FACE ( 'NONE', ( #14725, #629 ), #6706, .F. ) ;
#16660=CARTESIAN_POINT ( 'NONE',  ( 11.46874999795161543, -2.444050593749961031, -4.233219804643904460 ) ) ;
#16672=CARTESIAN_POINT ( 'NONE',  ( 8.343749997951613651, 2.246813503491833508, -4.409619785863906571 ) ) ;
#16682=VECTOR ( 'NONE', #1011, 1000.000000000000000 ) ;
#16689=EDGE_CURVE ( 'NONE', #17179, #2660, #19307, .T. ) ;
#16690=DIRECTION ( 'NONE',  ( 0.000000000000000000, 0.000000000000000000, 1.000000000000000000 ) ) ;
#16704=CARTESIAN_POINT ( 'NONE',  ( 11.81249999590322552, -2.068159791354221344, 5.387740456496221242 ) ) ;
#16708=CIRCLE ( 'NONE', #12508, 4.400000000000000355 ) ;
#16721=FACE_OUTER_BOUND ( 'NONE', #7937, .T. ) ;
#16722=CARTESIAN_POINT ( 'NONE',  ( 9.843749997951615427, 3.954556930911862000, -2.873153789725825469 ) ) ;
#16724=AXIS2_PLACEMENT_3D ( 'NONE', #17428, #9833, #6230 ) ;
#16732=DIRECTION ( 'NONE',  ( -1.000000000000000000, -0.000000000000000000, -0.000000000000000000 ) ) ;
#16737=CARTESIAN_POINT ( 'NONE',  ( 10.34374999795161543, 4.150607464521792522, 2.695436003842732298 ) ) ;
#16744=VERTEX_POINT ( 'NONE', #18028 ) ;
#16749=FACE_OUTER_BOUND ( 'NONE', #5598, .T. ) ;
#16753=STYLED_ITEM ( 'NONE', ( #6166 ), #7808 ) ;
#16755=ADVANCED_FACE ( 'NONE', ( #16721 ), #10421, .F. ) ;
#16782=VERTEX_POINT ( 'NONE', #11005 ) ;
#16788=CARTESIAN_POINT ( 'NONE',  ( 12.34374999795161543, 4.888101187500000222, 0.7741991708318884946 ) ) ;
#16790=ADVANCED_FACE ( 'NONE', ( #14205 ), #11778, .F. ) ;
#16804=CARTESIAN_POINT ( 'NONE',  ( 12.99999999999999467, 4.471046188018904743, 1.976722499206014838 ) ) ;
#16815=CARTESIAN_POINT ( 'NONE',  ( 6.468749997951615427, -4.233219804643852946, -2.444050593750049849 ) ) ;
#16818=CARTESIAN_POINT ( 'NONE',  ( 11.00000000000000711, 5.700000000000001066, -3.490243377569957047E-16 ) ) ;
#16822=ORIENTED_EDGE ( 'NONE', *, *, #1148, .T. ) ;
#16824=DIRECTION ( 'NONE',  ( 0.000000000000000000, -0.7315216790650488354, -0.6818181818181821008 ) ) ;
#16825=CARTESIAN_POINT ( 'NONE',  ( 12.46874999795161543, 1.016293382781411792, 4.781284448697194378 ) ) ;
#16832=CARTESIAN_POINT ( 'NONE',  ( 6.468749997951615427, -3.413342815706642518E-14, 4.888101187500000222 ) ) ;
#16835=CARTESIAN_POINT ( 'NONE',  ( 5.500000000000005329, 0.000000000000000000, 0.000000000000000000 ) ) ;
#16842=ORIENTED_EDGE ( 'NONE', *, *, #16041, .T. ) ;
#16861=CARTESIAN_POINT ( 'NONE',  ( 7.000000000000005329, -5.575441324182703440, 1.185096637661176677 ) ) ;
#16875=CARTESIAN_POINT ( 'NONE',  ( 12.92161831991541554, 4.611601942845662272, 1.625176344145936147 ) ) ;
#16883=DIRECTION ( 'NONE',  ( -1.000000000000000000, -0.000000000000000000, -0.000000000000000000 ) ) ;
#16886=ORIENTED_EDGE ( 'NONE', *, *, #914, .F. ) ;
#16888=( NAMED_UNIT ( * ) SI_UNIT ( $, .STERADIAN. ) SOLID_ANGLE_UNIT ( ) );
#16912=CARTESIAN_POINT ( 'NONE',  ( 6.500000000000005329, 0.9027913098498568933, -5.699999999999999289 ) ) ;
#16917=CARTESIAN_POINT ( 'NONE',  ( 12.46874999795161543, -3.632567103900546712, 3.270778111535314281 ) ) ;
#16927=CARTESIAN_POINT ( 'NONE',  ( 7.968749997951616315, -2.246813503491864150, 4.409619785863891472 ) ) ;
#16939=VERTEX_POINT ( 'NONE', #19588 ) ;
#16940=EDGE_CURVE ( 'NONE', #9700, #19560, #14798, .T. ) ;
#16948=CARTESIAN_POINT ( 'NONE',  ( 12.99999999999999467, 0.3329550909587259966, 4.877148943244128176 ) ) ;
#16959=CARTESIAN_POINT ( 'NONE',  ( 12.31249999590322552, 2.850000000000057820, -4.936344801571268093 ) ) ;
#16964=CYLINDRICAL_SURFACE ( 'NONE', #19572, 5.700000000000001954 ) ;
#16966=CARTESIAN_POINT ( 'NONE',  ( 8.468749997951615427, 4.861323657744407001, 0.5109457054261784537 ) ) ;
#16988=ORIENTED_EDGE ( 'NONE', *, *, #7480, .F. ) ;
#17000=CARTESIAN_POINT ( 'NONE',  ( 12.00000000000000533, 4.235925505221192822, -3.814044456245444081 ) ) ;
#17003=CARTESIAN_POINT ( 'NONE',  ( 10.84374999795161543, -3.632567103900500971, -3.270778111535363131 ) ) ;
#17014=CARTESIAN_POINT ( 'NONE',  ( 8.468749997951615427, 4.861323657744407001, 0.5109457054261784537 ) ) ;
#17020=CARTESIAN_POINT ( 'NONE',  ( 6.500000000000005329, -4.484949146646330931, -3.631840208645857437 ) ) ;
#17029=ORIENTED_EDGE ( 'NONE', *, *, #7104, .T. ) ;
#17049=( BOUNDED_CURVE ( )  B_SPLINE_CURVE ( 2, ( #16815, #4396, #13797, #3089, #94, #19495, #16606, #12304, #4491, #18401, #2887, #5783, #18015, #4298, #2787 ),
 .UNSPECIFIED., .F., .F. ) 
 B_SPLINE_CURVE_WITH_KNOTS ( ( 3, 2, 2, 2, 2, 2, 2, 3 ),
 ( 0.000000000000000000, 0.05000000000000000278, 0.1000000000000000056, 0.1499999999999999944, 0.2000000000000000111, 0.2500000000000000000, 0.2999999999999999889, 0.3265529187307101844 ),
 .UNSPECIFIED. ) 
 CURVE ( )  GEOMETRIC_REPRESENTATION_ITEM ( )  RATIONAL_B_SPLINE_CURVE ( ( 1.000000000000000000, 0.9876883405951377704, 1.000000000000000000, 0.9876883405951377704, 1.000000000000000000, 0.9876883405951377704, 1.000000000000000000, 0.9876883405951377704, 1.000000000000000000, 0.9876883405951377704, 1.000000000000000000, 0.9876883405951377704, 1.000000000000000000, 0.9934617901676502383, 0.9938679225082089896 ) ) 
 REPRESENTATION_ITEM ( '' )  );
#17058=CARTESIAN_POINT ( 'NONE',  ( 10.84374999795161543, 1.016293382781477961, -4.781284448697179279 ) ) ;
#17094=CARTESIAN_POINT ( 'NONE',  ( 10.84374999795161543, -4.648860486681964055, 1.510506337161829027 ) ) ;
#17096=CARTESIAN_POINT ( 'NONE',  ( 9.000000000000005329, -0.5958122406255588199, -5.668774803599165857 ) ) ;
#17109=DIRECTION ( 'NONE',  ( -0.000000000000000000, -0.7315216790650492795, -0.6818181818181815457 ) ) ;
#17119=CARTESIAN_POINT ( 'NONE',  ( 7.500000000000005329, -3.143139765844555900, -4.840010801796527318 ) ) ;
#17126=CARTESIAN_POINT ( 'NONE',  ( 10.50000000000000533, -2.068159791354220900, 5.387740456496221242 ) ) ;
#17143=CARTESIAN_POINT ( 'NONE',  ( 13.00000000000000178, -4.568735188514048140, -1.737869959597788672 ) ) ;
#17154=CARTESIAN_POINT ( 'NONE',  ( 9.312499995903225525, -2.318398865532001363, -5.207209108562852684 ) ) ;
#17158=ORIENTED_EDGE ( 'NONE', *, *, #12124, .F. ) ;
#17161=CARTESIAN_POINT ( 'NONE',  ( 13.84374999795161543, -0.5109457054261780096, 4.861323657744406113 ) ) ;
#17164=( BOUNDED_CURVE ( )  B_SPLINE_CURVE ( 2, ( #2559, #3870, #14780, #3676, #19370, #5661, #9993, #16093, #2372, #8487, #2175, #19175, #16192 ),
 .UNSPECIFIED., .F., .F. ) 
 B_SPLINE_CURVE_WITH_KNOTS ( ( 3, 2, 2, 2, 2, 2, 3 ),
 ( 0.000000000000000000, 0.05000000000000000278, 0.1000000000000000056, 0.1499999999999999944, 0.2000000000000000111, 0.2500000000000000000, 0.2843253191101273170 ),
 .UNSPECIFIED. ) 
 CURVE ( )  GEOMETRIC_REPRESENTATION_ITEM ( )  RATIONAL_B_SPLINE_CURVE ( ( 1.000000000000000000, 0.9876883405951377704, 1.000000000000000000, 0.9876883405951377704, 1.000000000000000000, 0.9876883405951377704, 1.000000000000000000, 0.9876883405951377704, 1.000000000000000000, 0.9876883405951377704, 1.000000000000000000, 0.9915479672430580482, 0.9947006833465674713 ) ) 
 REPRESENTATION_ITEM ( '' )  );
#17178=FACE_BOUND ( 'NONE', #13950, .T. ) ;
#17179=VERTEX_POINT ( 'NONE', #19545 ) ;
#17189=CARTESIAN_POINT ( 'NONE',  ( 10.96874999795161720, 1.773574444220790136, -4.620319390059805187 ) ) ;
#17200=CARTESIAN_POINT ( 'NONE',  ( 12.50000000000000533, 5.142044285764750811, 2.620002426024544029 ) ) ;
#17204=ORIENTED_EDGE ( 'NONE', *, *, #7480, .T. ) ;
#17207=CARTESIAN_POINT ( 'NONE',  ( 7.968749997951616315, 4.942249507334556924, -0.2590123213420971182 ) ) ;
#17215=CARTESIAN_POINT ( 'NONE',  ( 7.843749997951614539, -1.510506337161893864, 4.648860486681943627 ) ) ;
#17222=CARTESIAN_POINT ( 'NONE',  ( 12.65441706489329299, 5.700000000000001954, 0.6173595171471270016 ) ) ;
#17232=ORIENTED_EDGE ( 'NONE', *, *, #18777, .F. ) ;
#17235=CARTESIAN_POINT ( 'NONE',  ( 2.999999999999998224, -3.950217066951267064, 3.681818181818180769 ) ) ;
#17246=ORIENTED_EDGE ( 'NONE', *, *, #6311, .F. ) ;
#17247=CARTESIAN_POINT ( 'NONE',  ( 11.50000000000000355, -2.068159791354146293, -5.387740456496247887 ) ) ;
#17248=CARTESIAN_POINT ( 'NONE',  ( 12.34374999795161543, 3.114526743279308896, -3.846120219227901593 ) ) ;
#17255=CARTESIAN_POINT ( 'NONE',  ( 14.84374999795161543, -1.988169868018592856, 4.465502636338025688 ) ) ;
#17257=ORIENTED_EDGE ( 'NONE', *, *, #18874, .T. ) ;
#17258=EDGE_CURVE ( 'NONE', #18200, #14637, #10557, .T. ) ;
#17266=EDGE_LOOP ( 'NONE', ( #15487, #8882, #3284, #57 ) ) ;
#17269=( BOUNDED_SURFACE ( )  B_SPLINE_SURFACE ( 1, 2, ( 
 ( #3247, #8251, #15861, #9362, #1852, #12661, #6630, #11159, #3646, #12758, #10960, #15762, #1755, #4954, #17161, #346, #17255 ),
 ( #2144, #14155, #15465, #9465, #16966, #15659, #18853, #18653, #13959, #3452, #252, #12856, #7943, #1943, #6334, #15560, #654 ) ),
 .UNSPECIFIED., .F., .F., .F. ) 
 B_SPLINE_SURFACE_WITH_KNOTS ( ( 2, 2 ),
 ( 3, 2, 2, 2, 2, 2, 2, 2, 3 ),
 ( 0.000000000000000000, 1.000000000000000000 ),
 ( 0.000000000000000000, 0.05000000000000000278, 0.1000000000000000056, 0.1499999999999999944, 0.2000000000000000111, 0.2500000000000000000, 0.2999999999999999889, 0.3499999999999999778, 0.4000000000000000222 ),
 .UNSPECIFIED. ) 
 GEOMETRIC_REPRESENTATION_ITEM ( )  RATIONAL_B_SPLINE_SURFACE ( (
 ( 1.000000000000000000, 0.9876883405951377704, 1.000000000000000000, 0.9876883405951377704, 1.000000000000000000, 0.9876883405951377704, 1.000000000000000000, 0.9876883405951377704, 1.000000000000000000, 0.9876883405951377704, 1.000000000000000000, 0.9876883405951377704, 1.000000000000000000, 0.9876883405951377704, 1.000000000000000000, 0.9876883405951377704, 1.000000000000000000),
 ( 1.000000000000000000, 0.9876883405951377704, 1.000000000000000000, 0.9876883405951377704, 1.000000000000000000, 0.9876883405951377704, 1.000000000000000000, 0.9876883405951377704, 1.000000000000000000, 0.9876883405951377704, 1.000000000000000000, 0.9876883405951377704, 1.000000000000000000, 0.9876883405951377704, 1.000000000000000000, 0.9876883405951377704, 1.000000000000000000) ) ) 
 REPRESENTATION_ITEM ( '' )  SURFACE ( )  );
#17285=DIRECTION ( 'NONE',  ( -0.4999999999999977240, -0.7499999999999961142, -0.4330127018922284576 ) ) ;
#17286=LINE ( 'NONE', #3575, #7207 ) ;
#17309=FACE_OUTER_BOUND ( 'NONE', #3386, .T. ) ;
#17311=CARTESIAN_POINT ( 'NONE',  ( 11.31249999590322375, -5.421022142882388373, 1.761396867937162769 ) ) ;
#17320=CARTESIAN_POINT ( 'NONE',  ( 10.31249999590322552, 4.611396867937201272, -3.350375938067097437 ) ) ;
#17351=CARTESIAN_POINT ( 'NONE',  ( 7.343749997951615427, -3.846120219227901149, -3.114526743279308896 ) ) ;
#17357=CARTESIAN_POINT ( 'NONE',  ( 11.34374999795161543, -1.773574444220757274, 4.620319390059819398 ) ) ;
#17365=ORIENTED_EDGE ( 'NONE', *, *, #7750, .T. ) ;
#17388=DIRECTION ( 'NONE',  ( -0.4999999999999979461, 0.7500000000000021094, -0.4330127018922180770 ) ) ;
#17409=CARTESIAN_POINT ( 'NONE',  ( 12.00000000000000533, -4.235925505221167064, 3.814044456245474279 ) ) ;
#17418=CARTESIAN_POINT ( 'NONE',  ( 10.84374999795161543, -4.648860486681964055, 1.510506337161829027 ) ) ;
#17427=CARTESIAN_POINT ( 'NONE',  ( 6.234374998975811266, -4.584782303107616031, 2.647025296874957689 ) ) ;
#17428=CARTESIAN_POINT ( 'NONE',  ( 0.000000000000000000, 0.000000000000000000, 0.000000000000000000 ) ) ;
#17431=CARTESIAN_POINT ( 'NONE',  ( 11.96874999795161365, -4.888101187499994893, -0.7741991708319226895 ) ) ;
#17435=DIRECTION ( 'NONE',  ( 1.000000000000000000, 0.000000000000000000, 0.000000000000000000 ) ) ;
#17441=ORIENTED_EDGE ( 'NONE', *, *, #17857, .T. ) ;
#17446=CARTESIAN_POINT ( 'NONE',  ( 6.843749997951615427, -4.233219804643904460, 2.444050593749960587 ) ) ;
#17464=CARTESIAN_POINT ( 'NONE',  ( 13.00000000000000178, -1.070668164103420805, -5.063333171156729762 ) ) ;
#17466=VERTEX_POINT ( 'NONE', #2490 ) ;
#17482=EDGE_CURVE ( 'NONE', #9454, #4538, #9001, .T. ) ;
#17486=CARTESIAN_POINT ( 'NONE',  ( 11.84374999795161365, 2.444050593750049405, -4.233219804643852946 ) ) ;
#17489=CARTESIAN_POINT ( 'NONE',  ( 6.656249997951614539, -4.233219804643904460, 2.444050593749960587 ) ) ;
#17510=CARTESIAN_POINT ( 'NONE',  ( 14.31249999590322552, -4.611396867937178179, -3.350375938067128967 ) ) ;
#17512=ORIENTED_EDGE ( 'NONE', *, *, #8103, .F. ) ;
#17523=EDGE_CURVE ( 'NONE', #4538, #871, #1198, .T. ) ;
#17527=CARTESIAN_POINT ( 'NONE',  ( 13.46874999795161543, -3.954556930911842016, -2.873153789725852558 ) ) ;
#17539=CARTESIAN_POINT ( 'NONE',  ( 10.98069898359950258, -0.5990941410143687529, 5.700000000000001954 ) ) ;
#17546=ADVANCED_FACE ( 'NONE', ( #18207 ), #15525, .F. ) ;
#17558=DIRECTION ( 'NONE',  ( 0.000000000000000000, 0.000000000000000000, 1.000000000000000000 ) ) ;
#17559=ORIENTED_EDGE ( 'NONE', *, *, #4889, .F. ) ;
#17561=CARTESIAN_POINT ( 'NONE',  ( 11.81249999590322552, -5.700000000000006395, 0.9027913098498173694 ) ) ;
#17581=CARTESIAN_POINT ( 'NONE',  ( -0.000000000000000000, 0.000000000000000000, 0.000000000000000000 ) ) ;
#17584=CARTESIAN_POINT ( 'NONE',  ( 13.00000000000000178, -4.545788521379982683, -1.798195097860023628 ) ) ;
#17590=DIRECTION ( 'NONE',  ( 0.000000000000000000, 0.000000000000000000, 1.000000000000000000 ) ) ;
#17597=CARTESIAN_POINT ( 'NONE',  ( 9.312499995903225525, 5.668774803599156975, 0.5958122406256377568 ) ) ;
#17601=CARTESIAN_POINT ( 'NONE',  ( 10.46874999795161720, -3.632567103900500971, -3.270778111535363131 ) ) ;
#17624=DIRECTION ( 'NONE',  ( 0.000000000000000000, 0.000000000000000000, 1.000000000000000000 ) ) ;
#17657=CARTESIAN_POINT ( 'NONE',  ( 13.00000000000000000, -3.840809689102975710, 4.211671987713753396 ) ) ;
#17670=CARTESIAN_POINT ( 'NONE',  ( 6.000593838912648081, -0.002144393866035136480, 5.699999596629369059 ) ) ;
#17689=CARTESIAN_POINT ( 'NONE',  ( 11.84374999795161365, 2.444050593749991229, 4.233219804643887585 ) ) ;
#17696=FACE_OUTER_BOUND ( 'NONE', #9766, .T. ) ;
#17699=( GEOMETRIC_REPRESENTATION_CONTEXT ( 3 ) GLOBAL_UNCERTAINTY_ASSIGNED_CONTEXT ( ( #603 ) ) GLOBAL_UNIT_ASSIGNED_CONTEXT ( ( #7664, #9184, #7461 ) ) REPRESENTATION_CONTEXT ( 'NONE', 'WORKASPACE' ) );
#17717=EDGE_CURVE ( 'NONE', #18417, #2730, #7314, .T. ) ;
#17720=CARTESIAN_POINT ( 'NONE',  ( 10.31249999590322552, -5.207209108562803834, -2.318398865532109721 ) ) ;
#17738=CARTESIAN_POINT ( 'NONE',  ( 6.000000000000005329, 5.700000000000001954, 0.000000000000000000 ) ) ;
#17739=CARTESIAN_POINT ( 'NONE',  ( 6.968749997951614539, 0.7741991708318887166, -4.888101187500000222 ) ) ;
#17768=SURFACE_STYLE_FILL_AREA ( #2451 ) ;
#17777=DIRECTION ( 'NONE',  ( -1.000000000000000000, 0.000000000000000000, 0.000000000000000000 ) ) ;
#17780=CARTESIAN_POINT ( 'NONE',  ( 13.00000000000000178, -4.568735188514048140, -1.737869959597788672 ) ) ;
#17788=CARTESIAN_POINT ( 'NONE',  ( 13.00000000000000178, -0.7793280607714923036, -4.825575716215948496 ) ) ;
#17797=( BOUNDED_CURVE ( )  B_SPLINE_CURVE ( 2, ( #12491, #379, #18488, #3283, #10989, #6362, #6661, #9396, #17094, #3385, #8077, #12787, #9496, #15593, #15397 ),
 .UNSPECIFIED., .F., .F. ) 
 B_SPLINE_CURVE_WITH_KNOTS ( ( 3, 2, 2, 2, 2, 2, 2, 3 ),
 ( 0.000000000000000000, 0.05000000000000000278, 0.1000000000000000056, 0.1499999999999999944, 0.2000000000000000111, 0.2500000000000000000, 0.2999999999999999889, 0.3078686208676164604 ),
 .UNSPECIFIED. ) 
 CURVE ( )  GEOMETRIC_REPRESENTATION_ITEM ( )  RATIONAL_B_SPLINE_CURVE ( ( 1.000000000000000000, 0.9876883405951377704, 1.000000000000000000, 0.9876883405951377704, 1.000000000000000000, 0.9876883405951377704, 1.000000000000000000, 0.9876883405951377704, 1.000000000000000000, 0.9876883405951377704, 1.000000000000000000, 0.9876883405951377704, 1.000000000000000000, 0.9980624843978382899, 0.9967347918236166837 ) ) 
 REPRESENTATION_ITEM ( '' )  );
#17804=CARTESIAN_POINT ( 'NONE',  ( 13.00000000000000178, 0.000000000000000000, 0.000000000000000000 ) ) ;
#17831=CARTESIAN_POINT ( 'NONE',  ( 2.999999999999998224, -3.950217066951263956, -3.681818181818183877 ) ) ;
#17833=ORIENTED_EDGE ( 'NONE', *, *, #8191, .F. ) ;
#17840=VERTEX_POINT ( 'NONE', #8949 ) ;
#17842=CARTESIAN_POINT ( 'NONE',  ( 12.99999999999969624, 1.390454305316116246, 5.264438301130793363 ) ) ;
#17844=CARTESIAN_POINT ( 'NONE',  ( 6.468749997951615427, 4.233219804643871598, 2.444050593750020095 ) ) ;
#17857=EDGE_CURVE ( 'NONE', #18527, #8351, #14382, .T. ) ;
#17868=ORIENTED_EDGE ( 'NONE', *, *, #13159, .F. ) ;
#17883=CARTESIAN_POINT ( 'NONE',  ( 14.81249999590322552, 4.080749450109650844, 4.080749450109649956 ) ) ;
#17884=CARTESIAN_POINT ( 'NONE',  ( 12.92161831991541554, -0.8983569717628844264, -4.806352606718993670 ) ) ;
#17897=DIRECTION ( 'NONE',  ( 1.000000000000000000, 0.000000000000000000, 0.000000000000000000 ) ) ;
#17922=CARTESIAN_POINT ( 'NONE',  ( 8.968749997951611874, 3.499494075959816541, -3.499494075959816541 ) ) ;
#17924=CARTESIAN_POINT ( 'NONE',  ( 6.656249997951614539, -3.413342815706642518E-14, 4.888101187500000222 ) ) ;
#17939=CARTESIAN_POINT ( 'NONE',  ( 6.843749997951615427, 4.233219804643887585, -2.444050593749990785 ) ) ;
#17941=ORIENTED_EDGE ( 'NONE', *, *, #4373, .T. ) ;
#17968=CARTESIAN_POINT ( 'NONE',  ( 11.96874999795161365, -1.773574444220693325, -4.620319390059842490 ) ) ;
#17977=CARTESIAN_POINT ( 'NONE',  ( 11.46874999795161543, -2.444050593750019651, 4.233219804643871598 ) ) ;
#17989=CARTESIAN_POINT ( 'NONE',  ( 7.343749997951615427, 0.7741991708318887166, -4.888101187500000222 ) ) ;
#17993=FILL_AREA_STYLE_COLOUR ( '', #18347 ) ;
#18003=CARTESIAN_POINT ( 'NONE',  ( 6.234374998975811266, 4.584782303107598267, -2.647025296874989664 ) ) ;
#18012=CARTESIAN_POINT ( 'NONE',  ( 7.843749997951614539, 3.270778111535313837, 3.632567103900546712 ) ) ;
#18015=CARTESIAN_POINT ( 'NONE',  ( 12.46874999795161543, 3.632567103900569361, -3.270778111535288080 ) ) ;
#18022=CARTESIAN_POINT ( 'NONE',  ( 6.000000000000005329, -3.980288726281172656E-14, 5.700000000000001066 ) ) ;
#18028=CARTESIAN_POINT ( 'NONE',  ( 6.000000000000005329, 0.000000000000000000, 4.400000000000000355 ) ) ;
#18029=CARTESIAN_POINT ( 'NONE',  ( 11.46874999795161543, 4.888101187500000222, -2.993098736590125853E-16 ) ) ;
#18032=CLOSED_SHELL ( 'NONE', ( #3130, #4803, #18339, #6543, #1150, #16648, #11766, #14714, #8031, #10640, #10211, #16755, #2801, #5079, #11056, #3735, #1351, #16790, #16147, #10572, #3950, #2984, #9571, #15733, #8325, #8403, #10161, #13811, #17546, #9597, #8727, #10449, #10505, #6050, #7473, #13993, #4671, #10795, #19144, #16036, #3060, #18919, #15127, #8232, #6922, #4193, #3318 ) ) ;
#18035=DIRECTION ( 'NONE',  ( -1.000000000000000000, 0.000000000000000000, 0.000000000000000000 ) ) ;
#18038=B_SPLINE_CURVE_WITH_KNOTS ( 'NONE', 3,
 ( #15380, #9179, #8243, #12848, #9379, #15479, #5336, #18847, #2039, #1669 ),
 .UNSPECIFIED., .F., .F.,
 ( 4, 3, 3, 4 ),
 ( 0.000000000000000000, 0.0001875345074742635362, 0.0003808595644229699441, 0.0005744879655065563686 ),
 .UNSPECIFIED. ) ;
#18044=CARTESIAN_POINT ( 'NONE',  ( 11.46874999795161543, 4.888101187500000222, -2.993098736590125853E-16 ) ) ;
#18054=AXIS2_PLACEMENT_3D ( 'NONE', #5492, #14316, #13209 ) ;
#18055=CARTESIAN_POINT ( 'NONE',  ( 13.00000000000000178, 0.7156116249825889009, 4.835865888676774915 ) ) ;
#18059=CARTESIAN_POINT ( 'NONE',  ( 7.500000000000005329, 2.620002426024544029, -5.142044285764751699 ) ) ;
#18064=CARTESIAN_POINT ( 'NONE',  ( 13.00000000000000178, 0.000000000000000000, 0.000000000000000000 ) ) ;
#18073=CARTESIAN_POINT ( 'NONE',  ( 14.46874999795161720, -4.861323657744410554, 0.5109457054261454800 ) ) ;
#18106=CARTESIAN_POINT ( 'NONE',  ( 7.343749997951615427, -4.620319390059841602, 1.773574444220693103 ) ) ;
#18114=CARTESIAN_POINT ( 'NONE',  ( 7.000000000000005329, -1.761396867937238486, 5.421022142882364392 ) ) ;
#18147=CARTESIAN_POINT ( 'NONE',  ( 6.968749997951614539, -4.620319390059841602, 1.773574444220693103 ) ) ;
#18154=DIRECTION ( 'NONE',  ( -1.000000000000000000, -0.000000000000000000, -0.000000000000000000 ) ) ;
#18155=( BOUNDED_SURFACE ( )  B_SPLINE_SURFACE ( 1, 2, ( 
 ( #3645, #8348, #15761, #12855, #653, #3843, #12756, #5137, #11253, #17357, #6727, #18952, #9768, #2243, #15217, #13807, #6191 ),
 ( #17844, #4138, #10251, #1139, #18409, #11740, #7492, #18314, #15316, #19708, #104, #1037, #16917, #4703, #203, #13611, #9114 ) ),
 .UNSPECIFIED., .F., .F., .F. ) 
 B_SPLINE_SURFACE_WITH_KNOTS ( ( 2, 2 ),
 ( 3, 2, 2, 2, 2, 2, 2, 2, 3 ),
 ( 0.000000000000000000, 1.000000000000000000 ),
 ( 0.000000000000000000, 0.05000000000000000278, 0.1000000000000000056, 0.1499999999999999944, 0.2000000000000000111, 0.2500000000000000000, 0.2999999999999999889, 0.3499999999999999778, 0.4000000000000000222 ),
 .UNSPECIFIED. ) 
 GEOMETRIC_REPRESENTATION_ITEM ( )  RATIONAL_B_SPLINE_SURFACE ( (
 ( 1.000000000000000000, 0.9876883405951377704, 1.000000000000000000, 0.9876883405951377704, 1.000000000000000000, 0.9876883405951377704, 1.000000000000000000, 0.9876883405951377704, 1.000000000000000000, 0.9876883405951377704, 1.000000000000000000, 0.9876883405951377704, 1.000000000000000000, 0.9876883405951377704, 1.000000000000000000, 0.9876883405951377704, 1.000000000000000000),
 ( 1.000000000000000000, 0.9876883405951377704, 1.000000000000000000, 0.9876883405951377704, 1.000000000000000000, 0.9876883405951377704, 1.000000000000000000, 0.9876883405951377704, 1.000000000000000000, 0.9876883405951377704, 1.000000000000000000, 0.9876883405951377704, 1.000000000000000000, 0.9876883405951377704, 1.000000000000000000, 0.9876883405951377704, 1.000000000000000000) ) ) 
 REPRESENTATION_ITEM ( '' )  SURFACE ( )  );
#18174=DIRECTION ( 'NONE',  ( -1.000000000000000000, 0.000000000000000000, 0.000000000000000000 ) ) ;
#18200=VERTEX_POINT ( 'NONE', #17831 ) ;
#18204=CARTESIAN_POINT ( 'NONE',  ( 8.968749997951611874, -1.280903732194386579, -4.780397808154273953 ) ) ;
#18206=B_SPLINE_CURVE_WITH_KNOTS ( 'NONE', 3,
 ( #9985, #15146, #18250, #16456 ),
 .UNSPECIFIED., .F., .F.,
 ( 4, 4 ),
 ( 0.000000000000000000, 0.001125480700308659687 ),
 .UNSPECIFIED. ) ;
#18207=FACE_OUTER_BOUND ( 'NONE', #1270, .T. ) ;
#18208=AXIS2_PLACEMENT_3D ( 'NONE', #4749, #5138, #12458 ) ;
#18210=CARTESIAN_POINT ( 'NONE',  ( 6.000000000000005329, 4.936344801571308061, -2.849999999999988987 ) ) ;
#18228=DIRECTION ( 'NONE',  ( 0.000000000000000000, 0.000000000000000000, 1.000000000000000000 ) ) ;
#18237=CARTESIAN_POINT ( 'NONE',  ( 13.31249999590322730, 1.185096637661216201, 5.575441324182695446 ) ) ;
#18238=AXIS2_PLACEMENT_3D ( 'NONE', #19408, #5790, #1408 ) ;
#18248=CARTESIAN_POINT ( 'NONE',  ( 13.00000000000000533, 4.611396867937201272, 3.350375938067096548 ) ) ;
#18249=ORIENTED_EDGE ( 'NONE', *, *, #14387, .F. ) ;
#18250=CARTESIAN_POINT ( 'NONE',  ( 12.99999999999998757, -4.496303326521678301, 2.563255015864473130 ) ) ;
#18251=EDGE_CURVE ( 'NONE', #871, #11866, #13040, .T. ) ;
#18269=ORIENTED_EDGE ( 'NONE', *, *, #15075, .F. ) ;
#18270=CARTESIAN_POINT ( 'NONE',  ( 11.34374999795161543, 4.888101187500000222, -0.7741991708318890497 ) ) ;
#18278=CIRCLE ( 'NONE', #12204, 5.700000000000001954 ) ;
#18283=CARTESIAN_POINT ( 'NONE',  ( 10.84374999795161543, 4.648860486681953397, -1.510506337161861667 ) ) ;
#18293=VECTOR ( 'NONE', #8793, 1000.000000000000000 ) ;
#18302=DIRECTION ( 'NONE',  ( 1.000000000000000000, 0.000000000000000000, 0.000000000000000000 ) ) ;
#18304=CIRCLE ( 'NONE', #1370, 4.400000000000000355 ) ;
#18307=ORIENTED_EDGE ( 'NONE', *, *, #4044, .F. ) ;
#18314=CARTESIAN_POINT ( 'NONE',  ( 9.968749997951617203, -0.2590123213421313686, 4.942249507334556036 ) ) ;
#18323=CARTESIAN_POINT ( 'NONE',  ( 11.84374999795161365, -4.888101187500000222, -3.383411828340740850E-14 ) ) ;
#18331=CARTESIAN_POINT ( 'NONE',  ( 13.84374999795161543, -0.5109457054261775655, 4.861323657744407001 ) ) ;
#18339=ADVANCED_FACE ( 'NONE', ( #15027 ), #15718, .T. ) ;
#18344=CARTESIAN_POINT ( 'NONE',  ( 6.468749997951615427, 4.233219804643887585, -2.444050593749990341 ) ) ;
#18347=COLOUR_RGB ( '', 0.31764706, 0.68627451, 0.89019608) ;
#18348=VECTOR ( 'NONE', #9083, 1000.000000000000000 ) ;
#18358=ORIENTED_EDGE ( 'NONE', *, *, #9382, .F. ) ;
#18363=FACE_OUTER_BOUND ( 'NONE', #1878, .T. ) ;
#18364=CARTESIAN_POINT ( 'NONE',  ( 6.656249997951614539, -4.233219804643852946, -2.444050593750049849 ) ) ;
#18367=EDGE_CURVE ( 'NONE', #3069, #7195, #14759, .T. ) ;
#18377=LINE ( 'NONE', #9762, #13230 ) ;
#18385=VECTOR ( 'NONE', #3778, 1000.000000000000000 ) ;
#18396=CARTESIAN_POINT ( 'NONE',  ( 13.00000000000000533, 5.207209108562852684, -2.318398865532001363 ) ) ;
#18397=CARTESIAN_POINT ( 'NONE',  ( 9.343749997951615427, -4.780397808154247308, -1.280903732194487166 ) ) ;
#18401=CARTESIAN_POINT ( 'NONE',  ( 10.96874999795161720, 1.773574444220789914, -4.620319390059805187 ) ) ;
#18409=CARTESIAN_POINT ( 'NONE',  ( 8.468749997951615427, 1.988169868018562436, 4.465502636338039011 ) ) ;
#18410=CARTESIAN_POINT ( 'NONE',  ( 11.50000000000000355, 2.068159791354184041, 5.387740456496232788 ) ) ;
#18417=VERTEX_POINT ( 'NONE', #18520 ) ;
#18418=DIRECTION ( 'NONE',  ( 0.000000000000000000, -1.000000000000000000, 0.000000000000000000 ) ) ;
#18419=DIRECTION ( 'NONE',  ( 0.000000000000000000, 0.000000000000000000, 1.000000000000000000 ) ) ;
#18446=CARTESIAN_POINT ( 'NONE',  ( 12.99999999999969624, 3.863910152777037421, -3.836387901770561104 ) ) ;
#18465=EDGE_CURVE ( 'NONE', #6403, #8156, #3415, .T. ) ;
#18475=ORIENTED_EDGE ( 'NONE', *, *, #6140, .T. ) ;
#18486=VERTEX_POINT ( 'NONE', #15821 ) ;
#18487=CARTESIAN_POINT ( 'NONE',  ( 9.343749997951615427, -1.280903732194386579, -4.780397808154273953 ) ) ;
#18488=CARTESIAN_POINT ( 'NONE',  ( 7.843749997951614539, -1.510506337161893864, 4.648860486681943627 ) ) ;
#18515=CARTESIAN_POINT ( 'NONE',  ( 6.968749997951614539, -0.7741991708319229115, 4.888101187499994893 ) ) ;
#18520=CARTESIAN_POINT ( 'NONE',  ( 6.000000000000005329, 0.000000000000000000, -5.700000000000001066 ) ) ;
#18527=VERTEX_POINT ( 'NONE', #12624 ) ;
#18556=( BOUNDED_SURFACE ( )  B_SPLINE_SURFACE ( 1, 2, ( 
 ( #16631, #9130, #15236, #1427, #1527, #8929, #9028, #11830, #7403, #13328, #5814, #7612, #18237, #4515, #6011, #7508, #2911 ),
 ( #17939, #13726, #12232, #10632, #11930, #3016, #12134, #16737, #16335, #13423, #7303, #4327, #18, #19429, #18331, #19630, #13528 ) ),
 .UNSPECIFIED., .F., .F., .F. ) 
 B_SPLINE_SURFACE_WITH_KNOTS ( ( 2, 2 ),
 ( 3, 2, 2, 2, 2, 2, 2, 2, 3 ),
 ( 0.000000000000000000, 1.000000000000000000 ),
 ( 0.000000000000000000, 0.05000000000000000278, 0.1000000000000000056, 0.1499999999999999944, 0.2000000000000000111, 0.2500000000000000000, 0.2999999999999999889, 0.3499999999999999778, 0.4000000000000000222 ),
 .UNSPECIFIED. ) 
 GEOMETRIC_REPRESENTATION_ITEM ( )  RATIONAL_B_SPLINE_SURFACE ( (
 ( 1.000000000000000000, 0.9876883405951377704, 1.000000000000000000, 0.9876883405951377704, 1.000000000000000000, 0.9876883405951377704, 1.000000000000000000, 0.9876883405951377704, 1.000000000000000000, 0.9876883405951377704, 1.000000000000000000, 0.9876883405951377704, 1.000000000000000000, 0.9876883405951377704, 1.000000000000000000, 0.9876883405951377704, 1.000000000000000000),
 ( 1.000000000000000000, 0.9876883405951377704, 1.000000000000000000, 0.9876883405951377704, 1.000000000000000000, 0.9876883405951377704, 1.000000000000000000, 0.9876883405951377704, 1.000000000000000000, 0.9876883405951377704, 1.000000000000000000, 0.9876883405951377704, 1.000000000000000000, 0.9876883405951377704, 1.000000000000000000, 0.9876883405951377704, 1.000000000000000000) ) ) 
 REPRESENTATION_ITEM ( '' )  SURFACE ( )  );
#18575=VERTEX_POINT ( 'NONE', #11608 ) ;
#18584=ORIENTED_EDGE ( 'NONE', *, *, #16191, .T. ) ;
#18597=DIRECTION ( 'NONE',  ( 0.000000000000000000, 0.7315216790650492795, -0.6818181818181815457 ) ) ;
#18603=CARTESIAN_POINT ( 'NONE',  ( 13.96874999795161365, -1.280903732194453859, 4.780397808154257078 ) ) ;
#18608=CARTESIAN_POINT ( 'NONE',  ( -2.000000000000001776, 0.000000000000000000, 6.500000000000000000 ) ) ;
#18611=CARTESIAN_POINT ( 'NONE',  ( 10.00000000000000533, 1.185096637661293251, -5.575441324182679459 ) ) ;
#18623=EDGE_CURVE ( 'NONE', #18417, #18575, #3905, .T. ) ;
#18637=DIRECTION ( 'NONE',  ( -1.000000000000000000, -0.000000000000000000, -0.000000000000000000 ) ) ;
#18653=CARTESIAN_POINT ( 'NONE',  ( 9.968749997951617203, 4.150607464521791634, 2.695436003842732298 ) ) ;
#18657=VECTOR ( 'NONE', #15600, 1000.000000000000000 ) ;
#18662=CIRCLE ( 'NONE', #16123, 5.700000000000001954 ) ;
#18663=ORIENTED_EDGE ( 'NONE', *, *, #15814, .T. ) ;
#18668=( BOUNDED_SURFACE ( )  B_SPLINE_SURFACE ( 1, 2, ( 
 ( #4998, #4265, #11667, #2751, #5655, #5853, #11865, #2456, #13363, #2094, #17977, #19559, #6680, #13175, #10084, #12804, #18073 ),
 ( #8770, #14772, #11309, #10176, #18901, #14871, #1263, #7340, #19461, #13458, #1067, #1165, #17409, #964, #3694, #4365, #7239 ) ),
 .UNSPECIFIED., .F., .F., .F. ) 
 B_SPLINE_SURFACE_WITH_KNOTS ( ( 2, 2 ),
 ( 3, 2, 2, 2, 2, 2, 2, 2, 3 ),
 ( 0.000000000000000000, 1.000000000000000000 ),
 ( 0.000000000000000000, 0.05000000000000000278, 0.1000000000000000056, 0.1499999999999999944, 0.2000000000000000111, 0.2500000000000000000, 0.2999999999999999889, 0.3499999999999999778, 0.4000000000000000222 ),
 .UNSPECIFIED. ) 
 GEOMETRIC_REPRESENTATION_ITEM ( )  RATIONAL_B_SPLINE_SURFACE ( (
 ( 1.000000000000000000, 0.9876883405951377704, 1.000000000000000000, 0.9876883405951377704, 1.000000000000000000, 0.9876883405951377704, 1.000000000000000000, 0.9876883405951377704, 1.000000000000000000, 0.9876883405951377704, 1.000000000000000000, 0.9876883405951377704, 1.000000000000000000, 0.9876883405951377704, 1.000000000000000000, 0.9876883405951377704, 1.000000000000000000),
 ( 1.000000000000000000, 0.9876883405951377704, 1.000000000000000000, 0.9876883405951377704, 1.000000000000000000, 0.9876883405951377704, 1.000000000000000000, 0.9876883405951377704, 1.000000000000000000, 0.9876883405951377704, 1.000000000000000000, 0.9876883405951377704, 1.000000000000000000, 0.9876883405951377704, 1.000000000000000000, 0.9876883405951377704, 1.000000000000000000) ) ) 
 REPRESENTATION_ITEM ( '' )  SURFACE ( )  );
#18673=LINE ( 'NONE', #175, #15414 ) ;
#18675=B_SPLINE_CURVE_WITH_KNOTS ( 'NONE', 3,
 ( #14172, #15676, #17842, #1136 ),
 .UNSPECIFIED., .F., .F.,
 ( 4, 4 ),
 ( 0.000000000000000000, 0.001126652051248518355 ),
 .UNSPECIFIED. ) ;
#18682=CARTESIAN_POINT ( 'NONE',  ( 6.234374998975811266, 4.584782303107579615, 2.647025296875021638 ) ) ;
#18685=CARTESIAN_POINT ( 'NONE',  ( 11.96874999795161365, 3.114526743279308896, -3.846120219227901593 ) ) ;
#18705=CARTESIAN_POINT ( 'NONE',  ( 8.468749997951615427, -2.873153789725853002, 3.954556930911842016 ) ) ;
#18706=EDGE_CURVE ( 'NONE', #15548, #3069, #9987, .T. ) ;
#18715=EDGE_CURVE ( 'NONE', #15581, #10033, #9020, .T. ) ;
#18716=ORIENTED_EDGE ( 'NONE', *, *, #10080, .F. ) ;
#18732=DIRECTION ( 'NONE',  ( 0.000000000000000000, 0.000000000000000000, 1.000000000000000000 ) ) ;
#18743=ORIENTED_EDGE ( 'NONE', *, *, #8191, .T. ) ;
#18744=CARTESIAN_POINT ( 'NONE',  ( 10.00000000000000533, -4.235925505221111997, -3.814044456245531567 ) ) ;
#18748=VERTEX_POINT ( 'NONE', #2686 ) ;
#18753=ORIENTED_EDGE ( 'NONE', *, *, #12718, .T. ) ;
#18758=ORIENTED_EDGE ( 'NONE', *, *, #19473, .T. ) ;
#18767=FACE_OUTER_BOUND ( 'NONE', #7506, .T. ) ;
#18771=EDGE_CURVE ( 'NONE', #18915, #7834, #1347, .T. ) ;
#18775=CARTESIAN_POINT ( 'NONE',  ( 12.99999999999999467, 4.021726346896418391, -2.778353902928511587 ) ) ;
#18777=EDGE_CURVE ( 'NONE', #16782, #18923, #17049, .T. ) ;
#18782=CARTESIAN_POINT ( 'NONE',  ( 10.34374999795161543, 0.2590123213421660631, -4.942249507334553371 ) ) ;
#18783=CARTESIAN_POINT ( 'NONE',  ( -2.000000000000001776, 0.000000000000000000, 0.000000000000000000 ) ) ;
#18787=CARTESIAN_POINT ( 'NONE',  ( 12.34374999795161543, -1.773574444220693325, -4.620319390059841602 ) ) ;
#18791=CARTESIAN_POINT ( 'NONE',  ( 8.843749997951615427, 4.861323657744407001, 0.5109457054261780096 ) ) ;
#18801=CARTESIAN_POINT ( 'NONE',  ( 7.000000000000005329, 5.575441324182695446, -1.185096637661215091 ) ) ;
#18802=CARTESIAN_POINT ( 'NONE',  ( 12.99999999999969980, -3.863910152777011664, 3.836387901770588194 ) ) ;
#18812=ORIENTED_EDGE ( 'NONE', *, *, #6322, .F. ) ;
#18820=CARTESIAN_POINT ( 'NONE',  ( 7.078124996927420476, 0.000000000000000000, -5.294050593750000644 ) ) ;
#18824=CARTESIAN_POINT ( 'NONE',  ( 8.468749997951615427, -2.873153789725853002, 3.954556930911842016 ) ) ;
#18825=ORIENTED_EDGE ( 'NONE', *, *, #1148, .F. ) ;
#18846=CARTESIAN_POINT ( 'NONE',  ( 11.34374999795161543, 1.773574444220790136, -4.620319390059805187 ) ) ;
#18847=CARTESIAN_POINT ( 'NONE',  ( 13.00000000000000178, -0.6516788101670404343, -4.844895625238700987 ) ) ;
#18853=CARTESIAN_POINT ( 'NONE',  ( 9.468749997951615427, 4.465502636338023912, 1.988169868018593300 ) ) ;
#18857=CARTESIAN_POINT ( 'NONE',  ( 7.000000000000005329, 3.814044456245473835, 4.235925505221166176 ) ) ;
#18865=VERTEX_POINT ( 'NONE', #14088 ) ;
#18874=EDGE_CURVE ( 'NONE', #8156, #4149, #6464, .T. ) ;
#18876=( NAMED_UNIT ( * ) SI_UNIT ( $, .STERADIAN. ) SOLID_ANGLE_UNIT ( ) );
#18878=ORIENTED_EDGE ( 'NONE', *, *, #2688, .F. ) ;
#18880=CARTESIAN_POINT ( 'NONE',  ( 13.00000000000000178, 3.869963285057293145, -2.986818217332015024 ) ) ;
#18884=CARTESIAN_POINT ( 'NONE',  ( 6.234374998975811266, 4.584782303107598267, -2.647025296874989664 ) ) ;
#18888=CARTESIAN_POINT ( 'NONE',  ( 11.50000000000000355, 5.700000000000000178, 0.9027913098498565603 ) ) ;
#18890=CARTESIAN_POINT ( 'NONE',  ( -2.000000000000001776, 0.000000000000000000, 0.000000000000000000 ) ) ;
#18901=CARTESIAN_POINT ( 'NONE',  ( 8.000000000000005329, 2.318398865532038666, 5.207209108562838473 ) ) ;
#18902=CARTESIAN_POINT ( 'NONE',  ( 14.34374999795161365, 1.280903732194486722, -4.780397808154247308 ) ) ;
#18905=ORIENTED_EDGE ( 'NONE', *, *, #174, .T. ) ;
#18911=AXIS2_PLACEMENT_3D ( 'NONE', #1297, #7582, #2991 ) ;
#18915=VERTEX_POINT ( 'NONE', #10798 ) ;
#18919=ADVANCED_FACE ( 'NONE', ( #3188 ), #9299, .T. ) ;
#18920=CIRCLE ( 'NONE', #11582, 5.700000000000001954 ) ;
#18923=VERTEX_POINT ( 'NONE', #12601 ) ;
#18952=CARTESIAN_POINT ( 'NONE',  ( 12.34374999795161543, -3.114526743279282250, 3.846120219227923798 ) ) ;
#18957=CARTESIAN_POINT ( 'NONE',  ( 8.312499995903225525, -1.761396867937238486, 5.421022142882364392 ) ) ;
#18966=DIRECTION ( 'NONE',  ( 0.000000000000000000, -0.8660254037844363761, -0.5000000000000039968 ) ) ;
#18967=CARTESIAN_POINT ( 'NONE',  ( 7.500000000000005329, -2.620002426024580000, 5.142044285764733935 ) ) ;
#18973=CARTESIAN_POINT ( 'NONE',  ( 13.00000000000000000, -4.333424887442987483, -2.261628166637620119 ) ) ;
#18982=CARTESIAN_POINT ( 'NONE',  ( 9.968749997951617203, 0.2590123213421660631, -4.942249507334553371 ) ) ;
#18983=CARTESIAN_POINT ( 'NONE',  ( 12.92161831991541554, 3.713244971082770629, -3.181176262573004898 ) ) ;
#18989=CARTESIAN_POINT ( 'NONE',  ( 9.500000000000005329, 5.142044285764750811, -2.620002426024544473 ) ) ;
#18992=DIRECTION ( 'NONE',  ( 1.000000000000000000, 0.000000000000000000, 0.000000000000000000 ) ) ;
#19001=DIRECTION ( 'NONE',  ( 0.000000000000000000, 0.000000000000000000, 1.000000000000000000 ) ) ;
#19005=CARTESIAN_POINT ( 'NONE',  ( 6.843749997951615427, -4.233219804643904460, 2.444050593749960587 ) ) ;
#19010=FACE_OUTER_BOUND ( 'NONE', #6931, .T. ) ;
#19016=CARTESIAN_POINT ( 'NONE',  ( 6.656249997951614539, 0.000000000000000000, -5.700000000000001066 ) ) ;
#19023=CARTESIAN_POINT ( 'NONE',  ( 10.96874999795161720, -4.888101187500005551, 0.7741991708318548548 ) ) ;
#19048=DIRECTION ( 'NONE',  ( 0.000000000000000000, 0.000000000000000000, 1.000000000000000000 ) ) ;
#19050=CARTESIAN_POINT ( 'NONE',  ( 12.99999999999969624, -5.254364458093111701, -1.428050399360220490 ) ) ;
#19052=LINE ( 'NONE', #10061, #16352 ) ;
#19062=CARTESIAN_POINT ( 'NONE',  ( 13.00000000000000533, -0.2990843904630008931, 5.438532396800195734 ) ) ;
#19063=CARTESIAN_POINT ( 'NONE',  ( 9.500000000000005329, -5.142044285764769462, 2.620002426024508502 ) ) ;
#19076=ORIENTED_EDGE ( 'NONE', *, *, #1247, .F. ) ;
#19078=( BOUNDED_CURVE ( )  B_SPLINE_CURVE ( 2, ( #17670, #5548, #863, #18967, #16175, #9783, #11373, #19063, #14271, #12870, #14371, #14480, #6846, #9977, #2445 ),
 .UNSPECIFIED., .F., .F. ) 
 B_SPLINE_CURVE_WITH_KNOTS ( ( 3, 2, 2, 2, 2, 2, 2, 3 ),
 ( 0.000000000000000000, 0.04999999999999999584, 0.09999999999999999167, 0.1499999999999999944, 0.1999999999999999833, 0.2500000000000000000, 0.2999999999999999889, 0.3499999999999999778 ),
 .UNSPECIFIED. ) 
 CURVE ( )  GEOMETRIC_REPRESENTATION_ITEM ( )  RATIONAL_B_SPLINE_CURVE ( ( 1.000000000000000000, 0.9876883405951377704, 1.000000000000000000, 0.9876883405951377704, 1.000000000000000000, 0.9876883405951377704, 1.000000000000000000, 0.9876883405951377704, 1.000000000000000000, 0.9876883405951377704, 1.000000000000000000, 0.9876883405951377704, 1.000000000000000000, 0.9876883405951377704, 1.000000000000000000 ) ) 
 REPRESENTATION_ITEM ( '' )  );
#19079=CARTESIAN_POINT ( 'NONE',  ( 13.00000000000000178, 3.789407127742559833, -3.087705756618140285 ) ) ;
#19086=CARTESIAN_POINT ( 'NONE',  ( 6.843749997951615427, -4.233219804643904460, 2.444050593749960587 ) ) ;
#19088=CARTESIAN_POINT ( 'NONE',  ( 13.00000000000000000, 4.333424887443004359, 2.261628166637590365 ) ) ;
#19097=CARTESIAN_POINT ( 'NONE',  ( 10.96874999795161720, -3.114526743279228072, -3.846120219227966430 ) ) ;
#19102=CARTESIAN_POINT ( 'NONE',  ( 9.812499995903223748, -4.080749450109678378, 4.080749450109621534 ) ) ;
#19116=ORIENTED_EDGE ( 'NONE', *, *, #8, .T. ) ;
#19126=FACE_OUTER_BOUND ( 'NONE', #6468, .T. ) ;
#19140=DIRECTION ( 'NONE',  ( 1.000000000000000000, 0.000000000000000000, 0.000000000000000000 ) ) ;
#19144=ADVANCED_FACE ( 'NONE', ( #9081 ), #8976, .T. ) ;
#19149=DIRECTION ( 'NONE',  ( 0.000000000000000000, 0.7315216790650493905, -0.6818181818181815457 ) ) ;
#19151=CARTESIAN_POINT ( 'NONE',  ( -2.000000000000001776, 3.218695387886217230, 3.000000000000000000 ) ) ;
#19156=VECTOR ( 'NONE', #19755, 1000.000000000000000 ) ;
#19163=B_SPLINE_CURVE_WITH_KNOTS ( 'NONE', 3,
 ( #10839, #7625, #16948, #3228, #5830, #11943, #12047, #15144, #18055, #19644 ),
 .UNSPECIFIED., .F., .F.,
 ( 4, 3, 3, 4 ),
 ( 0.000000000000000000, 0.0001875345074742635904, 0.0003808595644229702693, 0.0005744879655065566939 ),
 .UNSPECIFIED. ) ;
#19164=( NAMED_UNIT ( * ) PLANE_ANGLE_UNIT ( ) SI_UNIT ( $, .RADIAN. ) );
#19167=ORIENTED_EDGE ( 'NONE', *, *, #18706, .F. ) ;
#19175=CARTESIAN_POINT ( 'NONE',  ( 12.65441706489329299, 3.384649025117562271, -4.627665042997699096 ) ) ;
#19180=CARTESIAN_POINT ( 'NONE',  ( 11.84374999795161365, -2.444050593749961031, -4.233219804643904460 ) ) ;
#19181=CARTESIAN_POINT ( 'NONE',  ( 7.312499995903225525, 4.936344801571289409, 2.850000000000024070 ) ) ;
#19190=( BOUNDED_SURFACE ( )  B_SPLINE_SURFACE ( 1, 2, ( 
 ( #6023, #18147, #10543, #4340, #10255, #13339, #19736, #3026, #13640, #2923, #1236, #8845, #11942, #5726, #14944, #9040, #1333 ),
 ( #5926, #15143, #7216, #2728, #1438, #1145, #12046, #11746, #7316, #13435, #10355, #7415, #13540, #16452, #19341, #14752, #7520 ) ),
 .UNSPECIFIED., .F., .F., .F. ) 
 B_SPLINE_SURFACE_WITH_KNOTS ( ( 2, 2 ),
 ( 3, 2, 2, 2, 2, 2, 2, 2, 3 ),
 ( 0.000000000000000000, 1.000000000000000000 ),
 ( 0.000000000000000000, 0.05000000000000000278, 0.1000000000000000056, 0.1499999999999999944, 0.2000000000000000111, 0.2500000000000000000, 0.2999999999999999889, 0.3499999999999999778, 0.4000000000000000222 ),
 .UNSPECIFIED. ) 
 GEOMETRIC_REPRESENTATION_ITEM ( )  RATIONAL_B_SPLINE_SURFACE ( (
 ( 1.000000000000000000, 0.9876883405951377704, 1.000000000000000000, 0.9876883405951377704, 1.000000000000000000, 0.9876883405951377704, 1.000000000000000000, 0.9876883405951377704, 1.000000000000000000, 0.9876883405951377704, 1.000000000000000000, 0.9876883405951377704, 1.000000000000000000, 0.9876883405951377704, 1.000000000000000000, 0.9876883405951377704, 1.000000000000000000),
 ( 1.000000000000000000, 0.9876883405951377704, 1.000000000000000000, 0.9876883405951377704, 1.000000000000000000, 0.9876883405951377704, 1.000000000000000000, 0.9876883405951377704, 1.000000000000000000, 0.9876883405951377704, 1.000000000000000000, 0.9876883405951377704, 1.000000000000000000, 0.9876883405951377704, 1.000000000000000000, 0.9876883405951377704, 1.000000000000000000) ) ) 
 REPRESENTATION_ITEM ( '' )  SURFACE ( )  );
#19196=CARTESIAN_POINT ( 'NONE',  ( 11.84374999795161365, -4.888101187500000222, -3.383411828340740850E-14 ) ) ;
#19210=CARTESIAN_POINT ( 'NONE',  ( 7.468749997951615427, -1.510506337161893864, 4.648860486681943627 ) ) ;
#19213=CARTESIAN_POINT ( 'NONE',  ( 10.81249999590322375, -4.840010801796461593, -3.143139765844656264 ) ) ;
#19243=EDGE_LOOP ( 'NONE', ( #17512, #14755, #18743, #18825, #9258, #12374, #3854, #10620 ) ) ;
#19245=CARTESIAN_POINT ( 'NONE',  ( 9.812499995903225525, -4.080749450109678378, 4.080749450109622423 ) ) ;
#19255=CARTESIAN_POINT ( 'NONE',  ( 6.234374998975811266, 4.584782303107579615, 2.647025296875021638 ) ) ;
#19264=CIRCLE ( 'NONE', #6463, 6.500000000000002665 ) ;
#19272=CARTESIAN_POINT ( 'NONE',  ( 8.843749997951615427, -1.988169868018530462, -4.465502636338051445 ) ) ;
#19279=CARTESIAN_POINT ( 'NONE',  ( 7.843749997951614539, -4.781284448697200595, 1.016293382781377819 ) ) ;
#19287=CARTESIAN_POINT ( 'NONE',  ( 6.656249997951614539, -4.936344801571327601, 2.849999999999954348 ) ) ;
#19294=ORIENTED_EDGE ( 'NONE', *, *, #12082, .F. ) ;
#19295=CARTESIAN_POINT ( 'NONE',  ( 15.31249999590322552, -5.668774803599162304, 0.5958122406255995651 ) ) ;
#19307=( BOUNDED_CURVE ( )  B_SPLINE_CURVE ( 2, ( #13613, #19614, #15117, #10516, #16614, #5995, #1114, #4211, #7188, #5901, #7493, #3001, #6093, #15218, #8814 ),
 .UNSPECIFIED., .F., .F. ) 
 B_SPLINE_CURVE_WITH_KNOTS ( ( 3, 2, 2, 2, 2, 2, 2, 3 ),
 ( 0.000000000000000000, 0.05000000000000000278, 0.1000000000000000056, 0.1499999999999999944, 0.2000000000000000111, 0.2500000000000000000, 0.2999999999999999889, 0.3265529187307101844 ),
 .UNSPECIFIED. ) 
 CURVE ( )  GEOMETRIC_REPRESENTATION_ITEM ( )  RATIONAL_B_SPLINE_CURVE ( ( 1.000000000000000000, 0.9876883405951377704, 1.000000000000000000, 0.9876883405951377704, 1.000000000000000000, 0.9876883405951377704, 1.000000000000000000, 0.9876883405951377704, 1.000000000000000000, 0.9876883405951377704, 1.000000000000000000, 0.9876883405951377704, 1.000000000000000000, 0.9934617901676502383, 0.9938679225082089896 ) ) 
 REPRESENTATION_ITEM ( '' )  );
#19308=CARTESIAN_POINT ( 'NONE',  ( 6.656249997951614539, 0.000000000000000000, -4.888101187500000222 ) ) ;
#19318=CARTESIAN_POINT ( 'NONE',  ( 6.000000000000005329, 5.388445916248354013E-16, -4.400000000000000355 ) ) ;
#19327=CARTESIAN_POINT ( 'NONE',  ( 13.00000000000000533, 4.859449410165161964, -2.460251518383709257 ) ) ;
#19341=CARTESIAN_POINT ( 'NONE',  ( 13.00000000000000533, 0.5958122406256767256, -5.668774803599153422 ) ) ;
#19342=PLANE ( 'NONE',  #2778 ) ;
#19351=LINE ( 'NONE', #3958, #6349 ) ;
#19354=EDGE_LOOP ( 'NONE', ( #12031, #16143, #2703, #752 ) ) ;
#19362=AXIS2_PLACEMENT_3D ( 'NONE', #17738, #19140, #14450 ) ;
#19365=CIRCLE ( 'NONE', #193, 5.400000000000000355 ) ;
#19370=CARTESIAN_POINT ( 'NONE',  ( 9.312499995903225525, -2.318398865532001363, -5.207209108562852684 ) ) ;
#19378=CARTESIAN_POINT ( 'NONE',  ( 14.84374999795161543, 2.873153789725825913, 3.954556930911861112 ) ) ;
#19388=LINE ( 'NONE', #4386, #15094 ) ;
#19397=CARTESIAN_POINT ( 'NONE',  ( 10.84374999795161543, -1.016293382781444654, 4.781284448697187273 ) ) ;
#19402=EDGE_LOOP ( 'NONE', ( #9407, #5943, #15840, #7679 ) ) ;
#19404=CARTESIAN_POINT ( 'NONE',  ( 8.468749997951615427, 2.873153789725825469, -3.954556930911862000 ) ) ;
#19408=CARTESIAN_POINT ( 'NONE',  ( 13.00000000000000178, 0.000000000000000000, 0.000000000000000000 ) ) ;
#19414=CARTESIAN_POINT ( 'NONE',  ( 7.343749997951615427, 0.7741991708318887166, -4.888101187500000222 ) ) ;
#19416=DIRECTION ( 'NONE',  ( -1.000000000000000000, -0.000000000000000000, -0.000000000000000000 ) ) ;
#19418=B_SPLINE_CURVE_WITH_KNOTS ( 'NONE', 3,
 ( #7109, #19327, #16630, #4227 ),
 .UNSPECIFIED., .F., .F.,
 ( 4, 4 ),
 ( 0.000000000000000000, 0.001125480700308659687 ),
 .UNSPECIFIED. ) ;
#19429=CARTESIAN_POINT ( 'NONE',  ( 13.34374999795161365, 0.2590123213420975623, 4.942249507334556924 ) ) ;
#19438=FACE_OUTER_BOUND ( 'NONE', #19243, .T. ) ;
#19453=CARTESIAN_POINT ( 'NONE',  ( 10.96874999795161720, -3.114526743279228072, -3.846120219227966430 ) ) ;
#19459=EDGE_CURVE ( 'NONE', #9124, #19695, #19078, .T. ) ;
#19461=CARTESIAN_POINT ( 'NONE',  ( 10.00000000000000533, -1.185096637661254171, 5.575441324182689229 ) ) ;
#19473=EDGE_CURVE ( 'NONE', #5140, #6183, #16267, .T. ) ;
#19475=CARTESIAN_POINT ( 'NONE',  ( 7.812499995903224637, 0.9027913098498568933, -5.699999999999999289 ) ) ;
#19479=VECTOR ( 'NONE', #6307, 1000.000000000000000 ) ;
#19494=CARTESIAN_POINT ( 'NONE',  ( 12.31249999590322552, -2.849999999999954792, -4.936344801571327601 ) ) ;
#19495=CARTESIAN_POINT ( 'NONE',  ( 8.968749997951613651, -1.280903732194386579, -4.780397808154273953 ) ) ;
#19502=ORIENTED_EDGE ( 'NONE', *, *, #14486, .T. ) ;
#19509=CARTESIAN_POINT ( 'NONE',  ( 13.00000000000000533, -4.611396867937178179, -3.350375938067128967 ) ) ;
#19513=FACE_OUTER_BOUND ( 'NONE', #17266, .T. ) ;
#19514=CARTESIAN_POINT ( 'NONE',  ( 12.65441706489329299, -3.384649025117529408, 4.627665042997723965 ) ) ;
#19522=CARTESIAN_POINT ( 'NONE',  ( -0.000000000000000000, 0.000000000000000000, 0.000000000000000000 ) ) ;
#19535=ORIENTED_EDGE ( 'NONE', *, *, #16689, .T. ) ;
#19540=( BOUNDED_CURVE ( )  B_SPLINE_CURVE ( 2, ( #4916, #11120, #8111, #17126, #5102, #6302, #8211, #11216, #5209 ),
 .UNSPECIFIED., .F., .F. ) 
 B_SPLINE_CURVE_WITH_KNOTS ( ( 3, 2, 2, 2, 3 ),
 ( 0.1666819079834116757, 0.2000000000000000111, 0.2500000000000000000, 0.2999999999999999889, 0.3499999999999999778 ),
 .UNSPECIFIED. ) 
 CURVE ( )  GEOMETRIC_REPRESENTATION_ITEM ( )  RATIONAL_B_SPLINE_CURVE ( ( 0.9945256517182512468, 0.9917959799814380917, 1.000000000000000000, 0.9876883405951377704, 1.000000000000000000, 0.9876883405951377704, 1.000000000000000000, 0.9876883405951377704, 1.000000000000000000 ) ) 
 REPRESENTATION_ITEM ( '' )  );
#19545=CARTESIAN_POINT ( 'NONE',  ( 6.468749997951615427, -3.413342815706642518E-14, 4.888101187500000222 ) ) ;
#19559=CARTESIAN_POINT ( 'NONE',  ( 11.96874999795161365, -3.114526743279282250, 3.846120219227923798 ) ) ;
#19560=VERTEX_POINT ( 'NONE', #4057 ) ;
#19567=VECTOR ( 'NONE', #14037, 1000.000000000000114 ) ;
#19572=AXIS2_PLACEMENT_3D ( 'NONE', #8038, #4656, #14154 ) ;
#19575=CARTESIAN_POINT ( 'NONE',  ( 10.81249999590322375, 5.142044285764749922, -2.620002426024544473 ) ) ;
#19579=DIRECTION ( 'NONE',  ( -0.4999999999999979461, -6.047423072554923456E-15, 0.8660254037844398178 ) ) ;
#19580=SURFACE_STYLE_FILL_AREA ( #7255 ) ;
#19584=DIRECTION ( 'NONE',  ( -0.4999999999999979461, 6.047423072554923456E-15, -0.8660254037844398178 ) ) ;
#19588=CARTESIAN_POINT ( 'NONE',  ( 13.00000000000000533, 5.207209108562852684, -2.318398865532001363 ) ) ;
#19596=CARTESIAN_POINT ( 'NONE',  ( 12.83455515208547482, -0.2987243419133426281, 5.700000000000001066 ) ) ;
#19612=EDGE_LOOP ( 'NONE', ( #939, #14852, #5250, #18249 ) ) ;
#19614=CARTESIAN_POINT ( 'NONE',  ( 6.968749997951614539, -0.7741991708319229115, 4.888101187499994893 ) ) ;
#19630=CARTESIAN_POINT ( 'NONE',  ( 14.34374999795161365, -1.280903732194453637, 4.780397808154257078 ) ) ;
#19644=CARTESIAN_POINT ( 'NONE',  ( 13.00000000000000178, 0.7793280607715257213, 4.825575716215943167 ) ) ;
#19645=EDGE_CURVE ( 'NONE', #15548, #18748, #19264, .T. ) ;
#19670=ORIENTED_EDGE ( 'NONE', *, *, #4418, .T. ) ;
#19675=CARTESIAN_POINT ( 'NONE',  ( 9.312499995903225525, 3.350375938067097437, -4.611396867937201272 ) ) ;
#19681=LINE ( 'NONE', #4473, #545 ) ;
#19690=CARTESIAN_POINT ( 'NONE',  ( 13.00000000000000000, 4.333424887443004359, 2.261628166637590365 ) ) ;
#19695=VERTEX_POINT ( 'NONE', #7328 ) ;
#19696=CARTESIAN_POINT ( 'NONE',  ( 6.468749997951615427, -4.233219804643852946, -2.444050593750049849 ) ) ;
#19700=CARTESIAN_POINT ( 'NONE',  ( 12.66727757604273386, -4.360680574150373717E-16, 5.700000000000001066 ) ) ;
#19708=CARTESIAN_POINT ( 'NONE',  ( 10.96874999795161720, -1.773574444220757274, 4.620319390059819398 ) ) ;
#19712=CARTESIAN_POINT ( 'NONE',  ( 11.96874999795161365, 4.888101187500000222, 0.7741991708318884946 ) ) ;
#19732=ORIENTED_EDGE ( 'NONE', *, *, #17523, .F. ) ;
#19736=CARTESIAN_POINT ( 'NONE',  ( 9.468749997951615427, -4.465502636338009701, -1.988169868018624609 ) ) ;
#19755=DIRECTION ( 'NONE',  ( -1.000000000000000000, 0.000000000000000000, 0.000000000000000000 ) ) ;
#19759=CARTESIAN_POINT ( 'NONE',  ( 9.343749997951615427, 3.499494075959816541, -3.499494075959816541 ) ) ;
#19763=ORIENTED_EDGE ( 'NONE', *, *, #18623, .T. ) ;
#19764=DIRECTION ( 'NONE',  ( 1.000000000000000000, 0.000000000000000000, 0.000000000000000000 ) ) ;
#19772=EDGE_LOOP ( 'NONE', ( #18716, #8454, #16127, #13347, #8361 ) ) ;
#19782=CARTESIAN_POINT ( 'NONE',  ( 13.34374999795161365, 4.409619785863906571, 2.246813503491833508 ) ) ;
ENDSEC;
END-ISO-10303-21;
